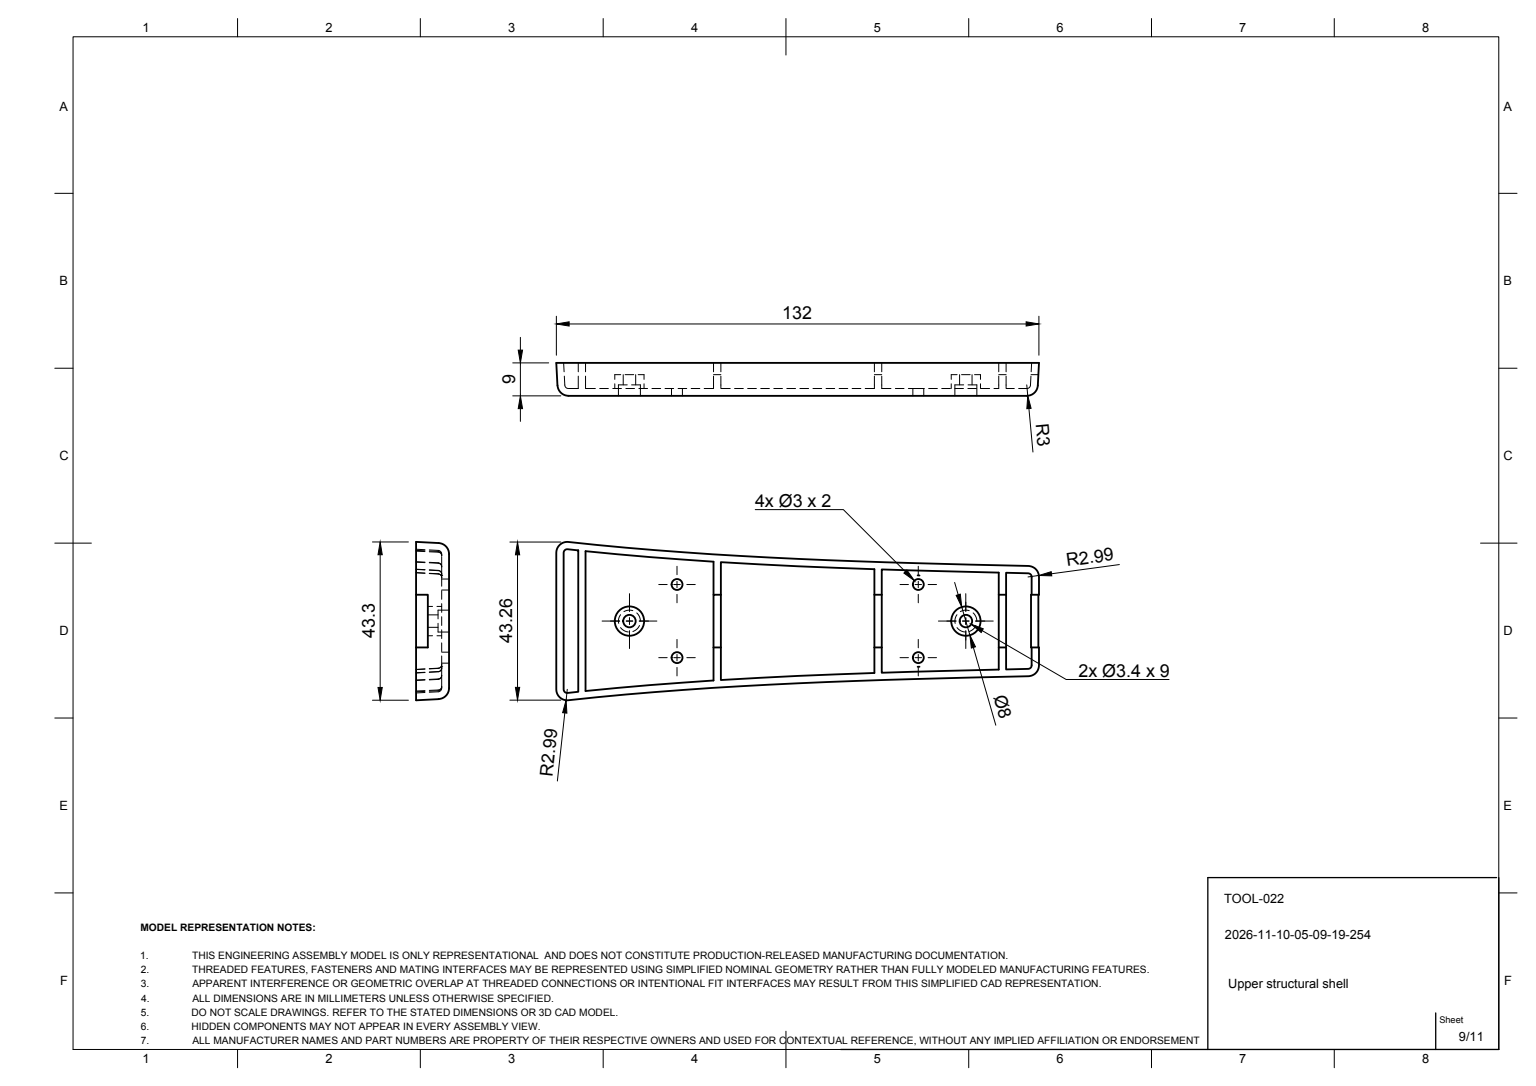
ISO-10303-21;
HEADER;
/* Generated by software containing ST-Developer
 * from STEP Tools, Inc. (www.steptools.com) 
 */

FILE_DESCRIPTION(
/* description */ (''),
/* implementation_level */ '2;1');

FILE_NAME(
/* name */ 'Upper structural shell.step',
/* time_stamp */ '2026-11-10T08:27:36-08:00',
/* author */ (''),
/* organization */ (''),
/* preprocessor_version */ 'ST-DEVELOPER v20.2',
/* originating_system */ 'Autodesk Translation Framework v15.17.0.0',
/* authorisation */ '');

FILE_SCHEMA (('AUTOMOTIVE_DESIGN { 1 0 10303 214 3 1 1 }'));
ENDSEC;

DATA;
#10=MECHANICAL_DESIGN_GEOMETRIC_PRESENTATION_REPRESENTATION('',(#570),#19090);
#76=SPHERICAL_SURFACE('',#7106,0.0999999999999999);
#77=SPHERICAL_SURFACE('',#7109,0.0999999999999997);
#78=SPHERICAL_SURFACE('',#7113,0.0999999999999998);
#79=SPHERICAL_SURFACE('',#7117,0.1);
#80=SPHERICAL_SURFACE('',#7122,0.3);
#81=SPHERICAL_SURFACE('',#7126,0.3);
#82=SPHERICAL_SURFACE('',#7130,0.3);
#83=SPHERICAL_SURFACE('',#7135,0.3);
#92=B_SPLINE_SURFACE_WITH_KNOTS('',3,3,((#10183,#10184,#10185,#10186),(#10187,
#10188,#10189,#10190),(#10191,#10192,#10193,#10194),(#10195,#10196,#10197,
#10198)),.UNSPECIFIED.,.F.,.F.,.F.,(4,4),(4,4),(0.0600191787356395,0.326709122771036),
(0.0105314009467253,0.683686938235975),.UNSPECIFIED.);
#93=B_SPLINE_SURFACE_WITH_KNOTS('',3,3,((#10203,#10204,#10205,#10206),(#10207,
#10208,#10209,#10210),(#10211,#10212,#10213,#10214),(#10215,#10216,#10217,
#10218)),.UNSPECIFIED.,.F.,.F.,.F.,(4,4),(4,4),(0.0251675824878611,0.0470055662028096),
(0.0103663370325175,0.682341693918943),.UNSPECIFIED.);
#94=B_SPLINE_SURFACE_WITH_KNOTS('',3,3,((#10228,#10229,#10230,#10231),(#10232,
#10233,#10234,#10235),(#10236,#10237,#10238,#10239),(#10240,#10241,#10242,
#10243),(#10244,#10245,#10246,#10247)),.UNSPECIFIED.,.F.,.F.,.F.,(4,1,4),
(4,4),(0.,0.571428571428571,1.),(0.796205213256333,4.31873271634551),
 .UNSPECIFIED.);
#95=B_SPLINE_SURFACE_WITH_KNOTS('',3,3,((#10252,#10253,#10254,#10255),(#10256,
#10257,#10258,#10259),(#10260,#10261,#10262,#10263),(#10264,#10265,#10266,
#10267),(#10268,#10269,#10270,#10271)),.UNSPECIFIED.,.F.,.F.,.F.,(4,1,4),
(4,4),(0.,0.571428571428571,1.),(0.335767855111383,0.605460332260614),
 .UNSPECIFIED.);
#96=B_SPLINE_SURFACE_WITH_KNOTS('',3,3,((#10290,#10291,#10292,#10293),(#10294,
#10295,#10296,#10297),(#10298,#10299,#10300,#10301),(#10302,#10303,#10304,
#10305),(#10306,#10307,#10308,#10309)),.UNSPECIFIED.,.F.,.F.,.F.,(4,1,4),
(4,4),(0.,0.571428571428571,1.),(8.8675541747208,12.3900816778099),
 .UNSPECIFIED.);
#97=B_SPLINE_SURFACE_WITH_KNOTS('',3,3,((#10314,#10315,#10316,#10317),(#10318,
#10319,#10320,#10321),(#10322,#10323,#10324,#10325),(#10326,#10327,#10328,
#10329)),.UNSPECIFIED.,.F.,.F.,.F.,(4,4),(4,4),(0.673290877228964,0.939980821264432),
(0.010531400969624,0.683686938235975),.UNSPECIFIED.);
#98=B_SPLINE_SURFACE_WITH_KNOTS('',3,3,((#10330,#10331,#10332,#10333),(#10334,
#10335,#10336,#10337),(#10338,#10339,#10340,#10341),(#10342,#10343,#10344,
#10345)),.UNSPECIFIED.,.F.,.F.,.F.,(4,4),(4,4),(0.952994433797115,0.974832417512139),
(0.0103663370325174,0.682341693895801),.UNSPECIFIED.);
#99=B_SPLINE_SURFACE_WITH_KNOTS('',3,3,((#10429,#10430,#10431,#10432),(#10433,
#10434,#10435,#10436),(#10437,#10438,#10439,#10440),(#10441,#10442,#10443,
#10444)),.UNSPECIFIED.,.F.,.F.,.F.,(4,4),(4,4),(0.341076481775573,0.660379921919131),
(0.0113804342297301,0.684288445414502),.UNSPECIFIED.);
#100=B_SPLINE_SURFACE_WITH_KNOTS('',3,3,((#10449,#10450,#10451,#10452),
(#10453,#10454,#10455,#10456),(#10457,#10458,#10459,#10460),(#10461,#10462,
#10463,#10464),(#10465,#10466,#10467,#10468)),.UNSPECIFIED.,.F.,.F.,.F.,
(4,1,4),(4,4),(0.,0.571428571428571,1.),(4.5128966022766,8.72381854299666),
 .UNSPECIFIED.);
#101=B_SPLINE_SURFACE_WITH_KNOTS('',3,3,((#10478,#10479,#10480,#10481),
(#10482,#10483,#10484,#10485),(#10486,#10487,#10488,#10489),(#10490,#10491,
#10492,#10493),(#10494,#10495,#10496,#10497)),.UNSPECIFIED.,.F.,.F.,.F.,
(4,1,4),(4,4),(0.,0.571428571428571,1.),(4.46246834806959,8.67339028878965),
 .UNSPECIFIED.);
#102=B_SPLINE_SURFACE_WITH_KNOTS('',3,3,((#10502,#10503,#10504,#10505),
(#10506,#10507,#10508,#10509),(#10510,#10511,#10512,#10513),(#10514,#10515,
#10516,#10517)),.UNSPECIFIED.,.F.,.F.,.F.,(4,4),(4,4),(0.33962007808087,
0.658923518224427),(0.0113804342297301,0.68428844541339),.UNSPECIFIED.);
#103=B_SPLINE_SURFACE_WITH_KNOTS('',3,3,((#10589,#10590,#10591,#10592),
(#10593,#10594,#10595,#10596),(#10597,#10598,#10599,#10600),(#10601,#10602,
#10603,#10604)),.UNSPECIFIED.,.F.,.F.,.F.,(4,4),(4,4),(0.67474627241906,
0.91907102854965),(0.0117551961069005,0.684448842095107),.UNSPECIFIED.);
#104=B_SPLINE_SURFACE_WITH_KNOTS('',3,3,((#10609,#10610,#10611,#10612),
(#10613,#10614,#10615,#10616),(#10617,#10618,#10619,#10620),(#10621,#10622,
#10623,#10624),(#10625,#10626,#10627,#10628)),.UNSPECIFIED.,.F.,.F.,.F.,
(4,1,4),(4,4),(0.,0.571428571428571,1.),(8.92068531110742,12.1251256661408),
 .UNSPECIFIED.);
#105=B_SPLINE_SURFACE_WITH_KNOTS('',3,3,((#10629,#10630,#10631,#10632),
(#10633,#10634,#10635,#10636),(#10637,#10638,#10639,#10640),(#10641,#10642,
#10643,#10644),(#10645,#10646,#10647,#10648)),.UNSPECIFIED.,.F.,.F.,.F.,
(4,1,4),(4,4),(0.,0.571428571428571,1.),(1.06116122492545,4.26560157995882),
 .UNSPECIFIED.);
#106=B_SPLINE_SURFACE_WITH_KNOTS('',3,3,((#10653,#10654,#10655,#10656),
(#10657,#10658,#10659,#10660),(#10661,#10662,#10663,#10664),(#10665,#10666,
#10667,#10668)),.UNSPECIFIED.,.F.,.F.,.F.,(4,4),(4,4),(0.0809289714503497,
0.325253727580939),(0.011755196108102,0.684448842095106),.UNSPECIFIED.);
#107=B_SPLINE_SURFACE_WITH_KNOTS('',3,3,((#10743,#10744,#10745,#10746),
(#10747,#10748,#10749,#10750),(#10751,#10752,#10753,#10754),(#10755,#10756,
#10757,#10758)),.UNSPECIFIED.,.F.,.F.,.F.,(4,4),(4,4),(0.932204931312898,
0.977820042778932),(0.0118590921259657,0.68448768567755),.UNSPECIFIED.);
#108=B_SPLINE_SURFACE_WITH_KNOTS('',3,3,((#10768,#10769,#10770,#10771),
(#10772,#10773,#10774,#10775),(#10776,#10777,#10778,#10779),(#10780,#10781,
#10782,#10783),(#10784,#10785,#10786,#10787)),.UNSPECIFIED.,.F.,.F.,.F.,
(4,1,4),(4,4),(0.,0.571428571428571,1.),(12.3228618033436,12.893479658151),
 .UNSPECIFIED.);
#109=B_SPLINE_SURFACE_WITH_KNOTS('',3,3,((#10801,#10802,#10803,#10804),
(#10805,#10806,#10807,#10808),(#10809,#10810,#10811,#10812),(#10813,#10814,
#10815,#10816)),.UNSPECIFIED.,.F.,.F.,.F.,(4,4),(4,4),(0.0221799572210682,
0.0677950686870383),(0.0118590921467069,0.68448768567755),.UNSPECIFIED.);
#110=B_SPLINE_SURFACE_WITH_KNOTS('',3,3,((#10826,#10827,#10828,#10829),
(#10830,#10831,#10832,#10833),(#10834,#10835,#10836,#10837),(#10838,#10839,
#10840,#10841),(#10842,#10843,#10844,#10845)),.UNSPECIFIED.,.F.,.F.,.F.,
(4,1,4),(4,4),(0.,0.571428571428571,1.),(0.29280723291527,0.863425087722636),
 .UNSPECIFIED.);
#111=B_SPLINE_SURFACE_WITH_KNOTS('',3,3,((#10859,#10860,#10861,#10862),
(#10863,#10864,#10865,#10866),(#10867,#10868,#10869,#10870),(#10871,#10872,
#10873,#10874),(#10875,#10876,#10877,#10878)),.UNSPECIFIED.,.F.,.F.,.F.,
(4,1,4),(4,4),(0.,0.571428571428571,1.),(0.00866835330220971,0.617725317592517),
 .UNSPECIFIED.);
#112=B_SPLINE_SURFACE_WITH_KNOTS('',3,3,((#10885,#10886,#10887,#10888),
(#10889,#10890,#10891,#10892),(#10893,#10894,#10895,#10896),(#10897,#10898,
#10899,#10900),(#10901,#10902,#10903,#10904),(#10905,#10906,#10907,#10908)),
 .UNSPECIFIED.,.F.,.F.,.F.,(4,1,1,4),(4,4),(0.,0.285714285714286,0.571428571428571,
1.),(0.00654045782928703,0.615688454110788),.UNSPECIFIED.);
#113=B_SPLINE_SURFACE_WITH_KNOTS('',3,3,((#10913,#10914,#10915,#10916),
(#10917,#10918,#10919,#10920),(#10921,#10922,#10923,#10924),(#10925,#10926,
#10927,#10928),(#10929,#10930,#10931,#10932),(#10933,#10934,#10935,#10936)),
 .UNSPECIFIED.,.F.,.F.,.F.,(4,1,1,4),(4,4),(0.,0.285714285714286,0.571428571428571,
1.),(0.00659363931523289,0.615688454110787),.UNSPECIFIED.);
#114=B_SPLINE_SURFACE_WITH_KNOTS('',3,3,((#10941,#10942,#10943,#10944),
(#10945,#10946,#10947,#10948),(#10949,#10950,#10951,#10952),(#10953,#10954,
#10955,#10956),(#10957,#10958,#10959,#10960)),.UNSPECIFIED.,.F.,.F.,.F.,
(4,1,4),(4,4),(0.,0.571428571428571,1.),(12.5808265588057,12.8505190359549),
 .UNSPECIFIED.);
#115=B_SPLINE_SURFACE_WITH_KNOTS('',3,3,((#10961,#10962,#10963,#10964),
(#10965,#10966,#10967,#10968),(#10969,#10970,#10971,#10972),(#10973,#10974,
#10975,#10976),(#10977,#10978,#10979,#10980)),.UNSPECIFIED.,.F.,.F.,.F.,
(4,1,4),(4,4),(0.,0.571428571428571,1.),(0.00865878607617127,0.617725317592517),
 .UNSPECIFIED.);
#116=B_SPLINE_SURFACE_WITH_KNOTS('',3,3,((#11006,#11007,#11008,#11009),
(#11010,#11011,#11012,#11013),(#11014,#11015,#11016,#11017),(#11018,#11019,
#11020,#11021),(#11022,#11023,#11024,#11025)),.UNSPECIFIED.,.F.,.F.,.F.,
(4,1,4),(4,4),(0.,0.571428571428571,1.),(-0.00615755989250974,0.617725317592517),
 .UNSPECIFIED.);
#117=B_SPLINE_SURFACE_WITH_KNOTS('',3,3,((#11044,#11045,#11046,#11047,#11048),
(#11049,#11050,#11051,#11052,#11053),(#11054,#11055,#11056,#11057,#11058),
(#11059,#11060,#11061,#11062,#11063),(#11064,#11065,#11066,#11067,#11068)),
 .UNSPECIFIED.,.F.,.F.,.F.,(4,1,4),(4,1,4),(0.,0.571428571428571,1.),(0.335767855111383,
5.71764434212835,12.893479658151),.UNSPECIFIED.);
#118=B_SPLINE_SURFACE_WITH_KNOTS('',3,3,((#11079,#11080,#11081,#11082),
(#11083,#11084,#11085,#11086),(#11087,#11088,#11089,#11090),(#11091,#11092,
#11093,#11094),(#11095,#11096,#11097,#11098),(#11099,#11100,#11101,#11102)),
 .UNSPECIFIED.,.F.,.F.,.F.,(4,1,1,4),(4,4),(0.,0.285714285714286,0.571428571428571,
1.),(-0.00844595120920508,0.615688454110788),.UNSPECIFIED.);
#119=B_SPLINE_SURFACE_WITH_KNOTS('',3,3,((#11111,#11112,#11113,#11114),
(#11115,#11116,#11117,#11118),(#11119,#11120,#11121,#11122),(#11123,#11124,
#11125,#11126),(#11127,#11128,#11129,#11130),(#11131,#11132,#11133,#11134)),
 .UNSPECIFIED.,.F.,.F.,.F.,(4,1,1,4),(4,4),(0.,0.285714285714286,0.571428571428571,
1.),(-0.00828643285111643,0.615688454110787),.UNSPECIFIED.);
#120=B_SPLINE_SURFACE_WITH_KNOTS('',3,3,((#11143,#11144,#11145,#11146,#11147),
(#11148,#11149,#11150,#11151,#11152),(#11153,#11154,#11155,#11156,#11157),
(#11158,#11159,#11160,#11161,#11162),(#11163,#11164,#11165,#11166,#11167)),
 .UNSPECIFIED.,.F.,.F.,.F.,(4,1,4),(4,1,4),(0.,0.571428571428571,1.),(0.29280723291527,
7.4686425489379,12.8505190359549),.UNSPECIFIED.);
#121=B_SPLINE_SURFACE_WITH_KNOTS('',3,3,((#11178,#11179,#11180,#11181),
(#11182,#11183,#11184,#11185),(#11186,#11187,#11188,#11189),(#11190,#11191,
#11192,#11193),(#11194,#11195,#11196,#11197)),.UNSPECIFIED.,.F.,.F.,.F.,
(4,1,4),(4,4),(0.,0.571428571428571,1.),(-0.0061862132014275,0.617725317592517),
 .UNSPECIFIED.);
#122=B_SPLINE_SURFACE_WITH_KNOTS('',3,3,((#11206,#11207,#11208,#11209),
(#11210,#11211,#11212,#11213),(#11214,#11215,#11216,#11217),(#11218,#11219,
#11220,#11221)),.UNSPECIFIED.,.F.,.F.,.F.,(4,4),(4,4),(0.025165545222094,
0.977821881680028),(0.,0.68448768567755),.UNSPECIFIED.);
#123=B_SPLINE_SURFACE_WITH_KNOTS('',3,3,((#11224,#11225,#11226,#11227),
(#11228,#11229,#11230,#11231),(#11232,#11233,#11234,#11235),(#11236,#11237,
#11238,#11239)),.UNSPECIFIED.,.F.,.F.,.F.,(4,4),(4,4),(0.0221781183199723,
0.974834454777906),(0.,0.68448768567755),.UNSPECIFIED.);
#172=B_SPLINE_CURVE_WITH_KNOTS('',3,(#9197,#9198,#9199,#9200),
 .UNSPECIFIED.,.F.,.F.,(4,4),(3.28016616408593,4.26236080300681),
 .UNSPECIFIED.);
#173=B_SPLINE_CURVE_WITH_KNOTS('',3,(#9204,#9205,#9206,#9207),
 .UNSPECIFIED.,.F.,.F.,(4,4),(8.92392608805945,9.90612072688831),
 .UNSPECIFIED.);
#174=B_SPLINE_CURVE_WITH_KNOTS('',3,(#9209,#9210,#9211,#9212,#9213,#9214,
#9215,#9216,#9217,#9218,#9219,#9220,#9221,#9222,#9223,#9224,#9225,#9226,
#9227),.UNSPECIFIED.,.F.,.F.,(4,3,3,3,3,3,4),(-0.050768112872884,-0.0388528786649772,
-0.0311058171716578,-0.0259830388669653,-0.0210744122964195,-0.0143837148934404,
0.),.UNSPECIFIED.);
#175=B_SPLINE_CURVE_WITH_KNOTS('',3,(#9229,#9230,#9231,#9232),
 .UNSPECIFIED.,.F.,.F.,(4,4),(9.9568018127159,12.1251256661408),
 .UNSPECIFIED.);
#176=B_SPLINE_CURVE_WITH_KNOTS('',3,(#9236,#9237,#9238,#9239),
 .UNSPECIFIED.,.F.,.F.,(4,4),(1.06116122492545,3.22948508825557),
 .UNSPECIFIED.);
#177=B_SPLINE_CURVE_WITH_KNOTS('',3,(#9240,#9241,#9242,#9243,#9244,#9245,
#9246,#9247,#9248,#9249,#9250,#9251,#9252,#9253,#9254,#9255,#9256,#9257,
#9258),.UNSPECIFIED.,.F.,.F.,(4,3,3,3,3,3,4),(-0.0507681129736439,-0.0388528772897764,
-0.0311058147321604,-0.0259830361493327,-0.0210744097201194,-0.0143837130754026,
-9.90506278315E-9),.UNSPECIFIED.);
#178=B_SPLINE_CURVE_WITH_KNOTS('',3,(#9406,#9407,#9408,#9409,#9410,#9411),
 .UNSPECIFIED.,.F.,.F.,(4,2,4),(-0.605566356596631,-0.303329629920269,-0.000148729590407126),
 .UNSPECIFIED.);
#179=B_SPLINE_CURVE_WITH_KNOTS('',3,(#9413,#9414,#9415,#9416,#9417,#9418,
#9419,#9420,#9421,#9422,#9423,#9424,#9425,#9426,#9427,#9428,#9429,#9430,
#9431,#9432,#9433,#9434,#9435,#9436,#9437,#9438,#9439,#9440),
 .UNSPECIFIED.,.F.,.F.,(4,3,3,3,3,3,3,3,3,4),(-0.153210533292091,-0.129383071834804,
-0.117098895005168,-0.0931297672424715,-0.0778761857300216,-0.065564095006876,
-0.0417435583396367,-0.038874550231651,-0.0150983388519663,0.),
 .UNSPECIFIED.);
#180=B_SPLINE_CURVE_WITH_KNOTS('',3,(#9444,#9445,#9446,#9447,#9448,#9449,
#9450,#9451,#9452,#9453,#9454,#9455,#9456,#9457,#9458,#9459,#9460,#9461,
#9462,#9463,#9464,#9465,#9466,#9467,#9468,#9469,#9470,#9471),
 .UNSPECIFIED.,.F.,.F.,(4,3,3,3,3,3,3,3,3,4),(-0.153244081227051,-0.129493605146206,
-0.117970006482883,-0.0941492904140308,-0.0876825809854227,-0.078828741443105,
-0.0548877675055393,-0.0394694906046094,-0.0155984926894347,0.),
 .UNSPECIFIED.);
#181=B_SPLINE_CURVE_WITH_KNOTS('',3,(#9472,#9473,#9474,#9475,#9476,#9477),
 .UNSPECIFIED.,.F.,.F.,(4,2,4),(-0.606539490527658,-0.303329031627741,-0.00112184825655631),
 .UNSPECIFIED.);
#182=B_SPLINE_CURVE_WITH_KNOTS('',3,(#9482,#9483,#9484,#9485,#9486,#9487),
 .UNSPECIFIED.,.F.,.F.,(4,2,4),(-0.606785247764818,-0.303663188081886,-0.00088649083675002),
 .UNSPECIFIED.);
#183=B_SPLINE_CURVE_WITH_KNOTS('',3,(#9489,#9490,#9491,#9492,#9493,#9494,
#9495,#9496,#9497,#9498,#9499,#9500,#9501,#9502,#9503,#9504,#9505,#9506,
#9507,#9508,#9509,#9510,#9511,#9512,#9513,#9514,#9515,#9516),
 .UNSPECIFIED.,.F.,.F.,(4,3,3,3,3,3,3,3,3,4),(-0.15258577077829,-0.128839317352572,
-0.117158786685373,-0.0932148261566644,-0.0780319390000633,-0.0653676349965338,
-0.0415665498371782,-0.0389909618069961,-0.0152059030050533,0.),
 .UNSPECIFIED.);
#184=B_SPLINE_CURVE_WITH_KNOTS('',3,(#9520,#9521,#9522,#9523,#9524,#9525,
#9526,#9527,#9528,#9529,#9530,#9531,#9532,#9533,#9534,#9535,#9536,#9537,
#9538,#9539,#9540,#9541,#9542,#9543,#9544,#9545,#9546,#9547),
 .UNSPECIFIED.,.F.,.F.,(4,3,3,3,3,3,3,3,3,4),(-0.152596853546747,-0.128825864440686,
-0.115507515430042,-0.0917263797372463,-0.0872428123353572,-0.0783995504057471,
-0.0544835945915644,-0.0392209901554083,-0.0154275313391792,0.),
 .UNSPECIFIED.);
#185=B_SPLINE_CURVE_WITH_KNOTS('',3,(#9549,#9550,#9551,#9552,#9553,#9554),
 .UNSPECIFIED.,.F.,.F.,(4,2,4),(-0.606440835737524,-0.303663090452391,-0.000542069086802599),
 .UNSPECIFIED.);
#186=B_SPLINE_CURVE_WITH_KNOTS('',3,(#9560,#9561,#9562,#9563,#9564,#9565),
 .UNSPECIFIED.,.F.,.F.,(4,2,4),(-0.607379220946441,-0.303761646676304,-0.00124422999587004),
 .UNSPECIFIED.);
#187=B_SPLINE_CURVE_WITH_KNOTS('',3,(#9567,#9568,#9569,#9570,#9571,#9572,
#9573,#9574,#9575,#9576,#9577,#9578,#9579,#9580,#9581,#9582,#9583,#9584,
#9585,#9586,#9587,#9588,#9589,#9590,#9591,#9592,#9593,#9594),
 .UNSPECIFIED.,.F.,.F.,(4,3,3,3,3,3,3,3,3,4),(-0.152287640102895,-0.128554450486317,
-0.115193035178751,-0.0912770810520543,-0.0781028969167454,-0.0652733399726575,
-0.0414820896655672,-0.0390446621366508,-0.0152552334863041,0.),
 .UNSPECIFIED.);
#188=B_SPLINE_CURVE_WITH_KNOTS('',3,(#9598,#9599,#9600,#9601,#9602,#9603,
#9604,#9605,#9606,#9607,#9608,#9609,#9610,#9611,#9612,#9613,#9614,#9615,
#9616,#9617,#9618,#9619,#9620,#9621,#9622,#9623,#9624,#9625),
 .UNSPECIFIED.,.F.,.F.,(4,3,3,3,3,3,3,3,3,4),(-0.152291020205185,-0.128517753946702,
-0.115248901231919,-0.0914807886786037,-0.0870359119466785,-0.0782017654295232,
-0.054298407767766,-0.03910658747416,-0.0153486482327859,0.),
 .UNSPECIFIED.);
#189=B_SPLINE_CURVE_WITH_KNOTS('',3,(#9627,#9628,#9629,#9630,#9631,#9632),
 .UNSPECIFIED.,.F.,.F.,(4,2,4),(-0.606279550122448,-0.303761677523001,-0.000144559171857295),
 .UNSPECIFIED.);
#190=B_SPLINE_CURVE_WITH_KNOTS('',3,(#9638,#9639,#9640,#9641,#9642,#9643),
 .UNSPECIFIED.,.F.,.F.,(4,2,4),(-0.607536685592867,-0.303784463250135,-0.00133982193348342),
 .UNSPECIFIED.);
#191=B_SPLINE_CURVE_WITH_KNOTS('',3,(#9644,#9645,#9646,#9647,#9648,#9649,
#9650,#9651,#9652,#9653,#9654,#9655,#9656,#9657,#9658,#9659,#9660,#9661,
#9662,#9663,#9664,#9665,#9666,#9667,#9668,#9669,#9670,#9671),
 .UNSPECIFIED.,.F.,.F.,(4,3,3,3,3,3,3,3,3,4),(-0.152217684890348,-0.128490376540845,
-0.11516578527262,-0.091253137134092,-0.0781160865160423,-0.0652495101170982,
-0.0414606291875136,-0.0390546905501479,-0.015263466236765,0.),
 .UNSPECIFIED.);
#192=B_SPLINE_CURVE_WITH_KNOTS('',3,(#9673,#9674,#9675,#9676,#9677,#9678,
#9679,#9680,#9681,#9682,#9683,#9684,#9685,#9686,#9687,#9688,#9689,#9690,
#9691,#9692,#9693,#9694,#9695,#9696,#9697,#9698,#9699,#9700),
 .UNSPECIFIED.,.F.,.F.,(4,3,3,3,3,3,3,3,3,4),(-0.152219351639196,-0.128444680332832,
-0.115193337419806,-0.0914284185691762,-0.0869890032859244,-0.0781648487722283,
-0.0542647883944502,-0.0390852411900305,-0.0153331469286526,0.),
 .UNSPECIFIED.);
#193=B_SPLINE_CURVE_WITH_KNOTS('',3,(#9702,#9703,#9704,#9705,#9706,#9707),
 .UNSPECIFIED.,.F.,.F.,(4,2,4),(-0.606231877025315,-0.303784501204342,-3.50089943914611E-5),
 .UNSPECIFIED.);
#194=B_SPLINE_CURVE_WITH_KNOTS('',3,(#9713,#9714,#9715,#9716),
 .UNSPECIFIED.,.F.,.F.,(4,4),(0.0108333608245492,0.617725317592517),
 .UNSPECIFIED.);
#195=B_SPLINE_CURVE_WITH_KNOTS('',3,(#9720,#9721,#9722,#9723),
 .UNSPECIFIED.,.F.,.F.,(4,4),(-0.617725317592517,-0.0108333608245492),
 .UNSPECIFIED.);
#196=B_SPLINE_CURVE_WITH_KNOTS('',3,(#9726,#9727,#9728,#9729),
 .UNSPECIFIED.,.F.,.F.,(4,4),(8.65483889175297,12.1899094612697),
 .UNSPECIFIED.);
#197=B_SPLINE_CURVE_WITH_KNOTS('',3,(#9730,#9731,#9732,#9733),
 .UNSPECIFIED.,.F.,.F.,(4,4),(0.491886782059505,4.00844302274363),
 .UNSPECIFIED.);
#198=B_SPLINE_CURVE_WITH_KNOTS('',3,(#9736,#9737,#9738,#9739,#9740,#9741,
#9742,#9743,#9744,#9745),.UNSPECIFIED.,.F.,.F.,(4,3,3,4),(4.20909064274042,
6.3236533433415,8.26419514194387,8.41669725637478),.UNSPECIFIED.);
#199=B_SPLINE_CURVE_WITH_KNOTS('',3,(#9748,#9749,#9750,#9751),
 .UNSPECIFIED.,.F.,.F.,(4,4),(8.61714174069208,11.8187712274298),
 .UNSPECIFIED.);
#200=B_SPLINE_CURVE_WITH_KNOTS('',3,(#9755,#9756,#9757,#9758),
 .UNSPECIFIED.,.F.,.F.,(4,4),(12.0182076143484,12.6179302061492),
 .UNSPECIFIED.);
#201=B_SPLINE_CURVE_WITH_KNOTS('',3,(#9759,#9760,#9761,#9762,#9763,#9764,
#9765,#9766,#9767,#9768,#9769,#9770,#9771,#9772,#9773,#9774,#9775,#9776,
#9777,#9778,#9779,#9780,#9781,#9782,#9783,#9784,#9785,#9786),
 .UNSPECIFIED.,.F.,.F.,(4,3,3,3,3,3,3,3,3,4),(0.,0.023812730958415,0.0390943730497349,
0.0628727645281949,0.0664866407211859,0.0780895647789142,0.102003044086093,
0.117056568347941,0.14081843048439,0.155095961761698),.UNSPECIFIED.);
#202=B_SPLINE_CURVE_WITH_KNOTS('',3,(#9790,#9791,#9792,#9793,#9794,#9795,
#9796,#9797,#9798,#9799,#9800,#9801,#9802,#9803,#9804,#9805,#9806,#9807,
#9808,#9809,#9810,#9811,#9812,#9813,#9814,#9815,#9816,#9817,#9818,#9819,
#9820,#9821,#9822,#9823,#9824,#9825,#9826),.UNSPECIFIED.,.F.,.F.,(4,3,3,
3,3,3,3,3,3,3,3,3,4),(0.,0.0535193130531386,0.107740084455895,0.117281563739951,
0.171478196787188,0.199460035548543,0.234266327019636,0.287962832542679,
0.34249270416273,0.351167719367162,0.408228095477446,0.46132246935065,0.46528847158773),
 .UNSPECIFIED.);
#203=B_SPLINE_CURVE_WITH_KNOTS('',3,(#9828,#9829,#9830,#9831),
 .UNSPECIFIED.,.F.,.F.,(4,4),(0.0221781183199723,0.974834454777906),
 .UNSPECIFIED.);
#204=B_SPLINE_CURVE_WITH_KNOTS('',3,(#9833,#9834,#9835,#9836,#9837,#9838,
#9839,#9840,#9841,#9842,#9843,#9844,#9845,#9846,#9847,#9848,#9849,#9850,
#9851,#9852,#9853,#9854,#9855,#9856,#9857,#9858,#9859,#9860,#9861,#9862,
#9863,#9864,#9865,#9866,#9867,#9868,#9869,#9870,#9871,#9872,#9873,#9874,
#9875),.UNSPECIFIED.,.F.,.F.,(4,3,3,3,3,3,3,3,3,3,3,3,3,3,4),(0.,0.0533317239385299,
0.107762434368039,0.117305236535198,0.171635266834242,0.216430402805854,
0.234303130921432,0.288010415584935,0.341932185058889,0.351200358601802,
0.360578786332496,0.414653942238971,0.427906071157934,0.482008506259547,
0.504658879840573),.UNSPECIFIED.);
#205=B_SPLINE_CURVE_WITH_KNOTS('',3,(#9879,#9880,#9881,#9882,#9883,#9884,
#9885,#9886,#9887,#9888,#9889,#9890,#9891,#9892,#9893,#9894,#9895,#9896,
#9897,#9898,#9899,#9900,#9901,#9902,#9903,#9904,#9905,#9906,#9907,#9908,
#9909,#9910,#9911,#9912,#9913,#9914,#9915,#9916,#9917,#9918,#9919,#9920,
#9921),.UNSPECIFIED.,.F.,.F.,(4,3,3,3,3,3,3,3,3,3,3,3,3,3,4),(0.,0.0533492049661439,
0.107791770949794,0.117401360885473,0.171729175646356,0.216477851539682,
0.234467324023732,0.288191829779795,0.342104640447882,0.351366010290958,
0.360619117109406,0.414688080797906,0.427993719046535,0.482081475021072,
0.504664253934307),.UNSPECIFIED.);
#206=B_SPLINE_CURVE_WITH_KNOTS('',3,(#9923,#9924,#9925,#9926),
 .UNSPECIFIED.,.F.,.F.,(4,4),(0.0251655452220943,0.977821881680028),
 .UNSPECIFIED.);
#207=B_SPLINE_CURVE_WITH_KNOTS('',3,(#9928,#9929,#9930,#9931,#9932,#9933,
#9934,#9935,#9936,#9937,#9938,#9939,#9940,#9941,#9942,#9943,#9944,#9945,
#9946,#9947,#9948,#9949,#9950,#9951,#9952,#9953,#9954,#9955,#9956,#9957,
#9958,#9959,#9960,#9961,#9962,#9963,#9964),.UNSPECIFIED.,.F.,.F.,(4,3,3,
3,3,3,3,3,3,3,3,3,4),(0.,0.053523079491772,0.107745541051727,0.117301531762597,
0.171497090450284,0.19946878868074,0.234298606923062,0.287998861062908,
0.34252758042597,0.351197710209308,0.408243668718811,0.4613343165756,0.465289627228313),
 .UNSPECIFIED.);
#208=B_SPLINE_CURVE_WITH_KNOTS('',3,(#9967,#9968,#9969,#9970,#9971,#9972,
#9973,#9974,#9975,#9976,#9977,#9978,#9979,#9980,#9981,#9982,#9983,#9984,
#9985,#9986,#9987,#9988,#9989,#9990,#9991,#9992,#9993,#9994),
 .UNSPECIFIED.,.F.,.F.,(4,3,3,3,3,3,3,3,3,4),(0.,0.0238139464176845,0.039101051769884,
0.0628789982206146,0.0664894862143964,0.0781003874493316,0.102014483019035,
0.11706667068295,0.140827139970411,0.155096347075245),.UNSPECIFIED.);
#209=B_SPLINE_CURVE_WITH_KNOTS('',3,(#9996,#9997,#9998,#9999),
 .UNSPECIFIED.,.F.,.F.,(4,4),(2.42791692093292E-5,0.602904494019558),
 .UNSPECIFIED.);
#210=B_SPLINE_CURVE_WITH_KNOTS('',3,(#10002,#10003,#10004,#10005),
 .UNSPECIFIED.,.F.,.F.,(4,4),(0.8033909285608,4.02187648095927),
 .UNSPECIFIED.);
#211=B_SPLINE_CURVE_WITH_KNOTS('',3,(#10008,#10009,#10010,#10011,#10012,
#10013,#10014,#10015,#10016,#10017),.UNSPECIFIED.,.F.,.F.,(4,3,3,4),(4.22337623295021,
6.17414866693447,6.32726315261627,8.45313487255185),.UNSPECIFIED.);
#212=B_SPLINE_CURVE_WITH_KNOTS('',3,(#10021,#10022,#10023,#10024),
 .UNSPECIFIED.,.F.,.F.,(4,4),(12.3921295467468,12.6843586902602),
 .UNSPECIFIED.);
#213=B_SPLINE_CURVE_WITH_KNOTS('',3,(#10026,#10027,#10028,#10029,#10030,
#10031,#10032,#10033,#10034,#10035,#10036,#10037,#10038,#10039,#10040,#10041,
#10042,#10043,#10044,#10045,#10046,#10047,#10048,#10049,#10050,#10051,#10052,
#10053,#10054,#10055,#10056,#10057,#10058,#10059),.UNSPECIFIED.,.F.,.F.,
(4,3,3,3,3,3,3,3,3,3,3,4),(0.,0.0238043957114055,0.0391346151758438,0.0629652053320384,
0.0721593756253901,0.0781571886687045,0.101948185591131,0.117123476992186,
0.12020682003633,0.142665945482357,0.166389927689249,0.168222194312373),
 .UNSPECIFIED.);
#214=B_SPLINE_CURVE_WITH_KNOTS('',3,(#10063,#10064,#10065,#10066,#10067,
#10068,#10069,#10070,#10071,#10072,#10073,#10074,#10075,#10076,#10077,#10078,
#10079,#10080,#10081,#10082,#10083,#10084,#10085,#10086,#10087,#10088,#10089,
#10090,#10091,#10092,#10093,#10094,#10095,#10096),.UNSPECIFIED.,.F.,.F.,
(4,3,3,3,3,3,3,3,3,3,3,4),(0.,0.023797882907907,0.039102479174454,0.0629340675289177,
0.0721439954475325,0.0781021576199648,0.101891255326939,0.117067721419617,
0.120193732390416,0.142636523050355,0.16636673084783,0.168220399847748),
 .UNSPECIFIED.);
#215=B_SPLINE_CURVE_WITH_KNOTS('',3,(#10098,#10099,#10100,#10101),
 .UNSPECIFIED.,.F.,.F.,(4,4),(2.71213177756024E-5,0.290725780256064),
 .UNSPECIFIED.);
#216=B_SPLINE_CURVE_WITH_KNOTS('',3,(#10111,#10112,#10113,#10114,#10115,
#10116),.UNSPECIFIED.,.F.,.F.,(4,2,4),(-0.6065913737563,-0.303324265158378,
-0.00121210420063977),.UNSPECIFIED.);
#217=B_SPLINE_CURVE_WITH_KNOTS('',3,(#10118,#10119,#10120,#10121,#10122,
#10123),.UNSPECIFIED.,.F.,.F.,(4,2,4),(-0.605468679705391,-0.303324901248498,
-8.9425867424664E-5),.UNSPECIFIED.);
#218=B_SPLINE_CURVE_WITH_KNOTS('',3,(#10125,#10126,#10127,#10128,#10129,
#10130,#10131,#10132,#10133,#10134,#10135,#10136,#10137,#10138,#10139,#10140,
#10141,#10142,#10143,#10144,#10145,#10146,#10147,#10148,#10149,#10150,#10151,
#10152),.UNSPECIFIED.,.F.,.F.,(4,3,3,3,3,3,3,3,3,4),(-0.153261590805415,
-0.129427422483982,-0.117093626371441,-0.093122524304512,-0.077863059046492,
-0.0655799937729104,-0.0417579003169496,-0.0388648221790391,-0.0150894148558222,
0.),.UNSPECIFIED.);
#219=B_SPLINE_CURVE_WITH_KNOTS('',3,(#10155,#10156,#10157,#10158,#10159,
#10160,#10161,#10162,#10163,#10164,#10165,#10166,#10167,#10168,#10169,#10170,
#10171,#10172,#10173,#10174,#10175,#10176,#10177,#10178,#10179,#10180,#10181,
#10182),.UNSPECIFIED.,.F.,.F.,(4,3,3,3,3,3,3,3,3,4),(-0.153296867786173,
-0.129546774976449,-0.118009772088948,-0.0941871764575653,-0.08771862273971,
-0.0788646444725944,-0.0549216410880561,-0.0394902966566095,-0.0156128557692252,
0.),.UNSPECIFIED.);
#220=B_SPLINE_CURVE_WITH_KNOTS('',3,(#10199,#10200,#10201,#10202),
 .UNSPECIFIED.,.F.,.F.,(4,4),(-4.3123055228435,-0.796205213256333),
 .UNSPECIFIED.);
#221=B_SPLINE_CURVE_WITH_KNOTS('',3,(#10220,#10221,#10222,#10223),
 .UNSPECIFIED.,.F.,.F.,(4,4),(-0.594853877716395,-0.335767855111383),
 .UNSPECIFIED.);
#222=B_SPLINE_CURVE_WITH_KNOTS('',3,(#10224,#10225,#10226,#10227),
 .UNSPECIFIED.,.F.,.F.,(4,4),(-0.615688454110788,-0.00935595183171186),
 .UNSPECIFIED.);
#223=B_SPLINE_CURVE_WITH_KNOTS('',3,(#10248,#10249,#10250,#10251),
 .UNSPECIFIED.,.F.,.F.,(4,4),(0.806548880270408,4.31873271634551),
 .UNSPECIFIED.);
#224=B_SPLINE_CURVE_WITH_KNOTS('',3,(#10273,#10274,#10275,#10276),
 .UNSPECIFIED.,.F.,.F.,(4,4),(0.335767855111383,0.605460332260614),
 .UNSPECIFIED.);
#225=B_SPLINE_CURVE_WITH_KNOTS('',3,(#10279,#10280,#10281,#10282),
 .UNSPECIFIED.,.F.,.F.,(4,4),(8.8675541747208,12.379738010796),
 .UNSPECIFIED.);
#226=B_SPLINE_CURVE_WITH_KNOTS('',3,(#10285,#10286,#10287,#10288),
 .UNSPECIFIED.,.F.,.F.,(4,4),(12.5808265588057,12.8505190359549),
 .UNSPECIFIED.);
#227=B_SPLINE_CURVE_WITH_KNOTS('',3,(#10310,#10311,#10312,#10313),
 .UNSPECIFIED.,.F.,.F.,(4,4),(-12.3900816778099,-8.87398136822274),
 .UNSPECIFIED.);
#228=B_SPLINE_CURVE_WITH_KNOTS('',3,(#10347,#10348,#10349,#10350),
 .UNSPECIFIED.,.F.,.F.,(4,4),(0.00935595183171174,0.615688454110787),
 .UNSPECIFIED.);
#229=B_SPLINE_CURVE_WITH_KNOTS('',3,(#10351,#10352,#10353,#10354),
 .UNSPECIFIED.,.F.,.F.,(4,4),(-12.8505190359549,-12.5914330133498),
 .UNSPECIFIED.);
#230=B_SPLINE_CURVE_WITH_KNOTS('',3,(#10357,#10358,#10359,#10360,#10361,
#10362),.UNSPECIFIED.,.F.,.F.,(4,2,4),(-0.606830654194234,-0.303665168982051,
-0.00091389508118378),.UNSPECIFIED.);
#231=B_SPLINE_CURVE_WITH_KNOTS('',3,(#10364,#10365,#10366,#10367,#10368,
#10369,#10370,#10371,#10372,#10373,#10374,#10375,#10376,#10377,#10378,#10379,
#10380,#10381,#10382,#10383,#10384,#10385,#10386,#10387,#10388,#10389,#10390,
#10391),.UNSPECIFIED.,.F.,.F.,(4,3,3,3,3,3,3,3,3,4),(-0.152562937837783,
-0.12881903955137,-0.117160811640917,-0.0932181166800446,-0.0780374575565173,
-0.0653603882662585,-0.0415602279441365,-0.0389951227734853,-0.0152093108541457,
0.),.UNSPECIFIED.);
#232=B_SPLINE_CURVE_WITH_KNOTS('',3,(#10395,#10396,#10397,#10398,#10399,
#10400,#10401,#10402,#10403,#10404,#10405,#10406,#10407,#10408,#10409,#10410,
#10411,#10412,#10413,#10414,#10415,#10416,#10417,#10418,#10419,#10420,#10421,
#10422),.UNSPECIFIED.,.F.,.F.,(4,3,3,3,3,3,3,3,3,4),(-0.152573286042523,
-0.128801685906155,-0.115487540236632,-0.091707628219999,-0.0872268515824704,
-0.07838422198738,-0.0544695788315335,-0.0392121213631617,-0.0154211067806385,
0.),.UNSPECIFIED.);
#233=B_SPLINE_CURVE_WITH_KNOTS('',3,(#10423,#10424,#10425,#10426,#10427,
#10428),.UNSPECIFIED.,.F.,.F.,(4,2,4),(-0.606417229744719,-0.30366508312326,
-0.000500462001714608),.UNSPECIFIED.);
#234=B_SPLINE_CURVE_WITH_KNOTS('',3,(#10445,#10446,#10447,#10448),
 .UNSPECIFIED.,.F.,.F.,(4,4),(-8.7204856127415,-4.5128966022766),
 .UNSPECIFIED.);
#235=B_SPLINE_CURVE_WITH_KNOTS('',3,(#10469,#10470,#10471,#10472),
 .UNSPECIFIED.,.F.,.F.,(4,4),(4.51913891174751,8.72381854299666),
 .UNSPECIFIED.);
#236=B_SPLINE_CURVE_WITH_KNOTS('',3,(#10474,#10475,#10476,#10477),
 .UNSPECIFIED.,.F.,.F.,(4,4),(4.46246834806959,8.66714797931881),
 .UNSPECIFIED.);
#237=B_SPLINE_CURVE_WITH_KNOTS('',3,(#10498,#10499,#10500,#10501),
 .UNSPECIFIED.,.F.,.F.,(4,4),(-8.67339028878965,-4.46580127832475),
 .UNSPECIFIED.);
#238=B_SPLINE_CURVE_WITH_KNOTS('',3,(#10520,#10521,#10522,#10523,#10524,
#10525),.UNSPECIFIED.,.F.,.F.,(4,2,4),(-0.607391644691745,-0.303762155877002,
-0.00125172564267001),.UNSPECIFIED.);
#239=B_SPLINE_CURVE_WITH_KNOTS('',3,(#10526,#10527,#10528,#10529,#10530,
#10531,#10532,#10533,#10534,#10535,#10536,#10537,#10538,#10539,#10540,#10541,
#10542,#10543,#10544,#10545,#10546,#10547,#10548,#10549,#10550,#10551,#10552,
#10553),.UNSPECIFIED.,.F.,.F.,(4,3,3,3,3,3,3,3,3,4),(-0.152281539067936,
-0.12854821222061,-0.115190816126163,-0.0912758856104041,-0.0781043161616985,
-0.0652713841318381,-0.0414808619979686,-0.039045740680325,-0.0152551599791835,
0.),.UNSPECIFIED.);
#240=B_SPLINE_CURVE_WITH_KNOTS('',3,(#10555,#10556,#10557,#10558,#10559,
#10560,#10561,#10562,#10563,#10564,#10565,#10566,#10567,#10568,#10569,#10570,
#10571,#10572,#10573,#10574,#10575,#10576,#10577,#10578,#10579,#10580,#10581,
#10582),.UNSPECIFIED.,.F.,.F.,(4,3,3,3,3,3,3,3,3,4),(-0.152284734818265,
-0.128510300097745,-0.115243636037359,-0.0914764658269932,-0.0870316758632336,
-0.078197793898112,-0.0542955901223581,-0.0391042908842167,-0.0153462458625635,
0.),.UNSPECIFIED.);
#241=B_SPLINE_CURVE_WITH_KNOTS('',3,(#10583,#10584,#10585,#10586,#10587,
#10588),.UNSPECIFIED.,.F.,.F.,(4,2,4),(-0.606273164239037,-0.303762187833104,
-0.000133245189939568),.UNSPECIFIED.);
#242=B_SPLINE_CURVE_WITH_KNOTS('',3,(#10605,#10606,#10607,#10608),
 .UNSPECIFIED.,.F.,.F.,(4,4),(-12.1227852464729,-8.92068531110742),
 .UNSPECIFIED.);
#243=B_SPLINE_CURVE_WITH_KNOTS('',3,(#10649,#10650,#10651,#10652),
 .UNSPECIFIED.,.F.,.F.,(4,4),(-4.26560157995882,-1.06350164459338),
 .UNSPECIFIED.);
#244=B_SPLINE_CURVE_WITH_KNOTS('',3,(#10671,#10672,#10673,#10674,#10675,
#10676),.UNSPECIFIED.,.F.,.F.,(4,2,4),(-0.607545900263938,-0.303784727094449,
-0.00134539382494125),.UNSPECIFIED.);
#245=B_SPLINE_CURVE_WITH_KNOTS('',3,(#10678,#10679,#10680,#10681,#10682,
#10683,#10684,#10685,#10686,#10687,#10688,#10689,#10690,#10691,#10692,#10693,
#10694,#10695,#10696,#10697,#10698,#10699,#10700,#10701,#10702,#10703,#10704,
#10705),.UNSPECIFIED.,.F.,.F.,(4,3,3,3,3,3,3,3,3,4),(-0.152214473108837,
-0.128485298747135,-0.115164309990209,-0.0912534321321267,-0.0781163092888813,
-0.0652482412471129,-0.0414606388666645,-0.0390548598067502,-0.0152611452145655,
0.),.UNSPECIFIED.);
#246=B_SPLINE_CURVE_WITH_KNOTS('',3,(#10709,#10710,#10711,#10712,#10713,
#10714,#10715,#10716,#10717,#10718,#10719,#10720,#10721,#10722,#10723,#10724,
#10725,#10726,#10727,#10728,#10729,#10730,#10731,#10732,#10733,#10734,#10735,
#10736),.UNSPECIFIED.,.F.,.F.,(4,3,3,3,3,3,3,3,3,4),(-0.152216110966007,
-0.128438825687404,-0.115191384846861,-0.0914281188167518,-0.0869870566155827,
-0.0781642271790374,-0.0542662950786889,-0.0390848818783988,-0.0153309789665,
0.),.UNSPECIFIED.);
#247=B_SPLINE_CURVE_WITH_KNOTS('',3,(#10737,#10738,#10739,#10740,#10741,
#10742),.UNSPECIFIED.,.F.,.F.,(4,2,4),(-0.606227037063105,-0.303784766192107,
-2.65251918123988E-5),.UNSPECIFIED.);
#248=B_SPLINE_CURVE_WITH_KNOTS('',3,(#10760,#10761,#10762,#10763),
 .UNSPECIFIED.,.F.,.F.,(4,4),(0.0107208554739345,0.617725317592517),
 .UNSPECIFIED.);
#249=B_SPLINE_CURVE_WITH_KNOTS('',3,(#10764,#10765,#10766,#10767),
 .UNSPECIFIED.,.F.,.F.,(4,4),(-12.893479658151,-12.3228618033436),
 .UNSPECIFIED.);
#250=B_SPLINE_CURVE_WITH_KNOTS('',3,(#10790,#10791,#10792,#10793),
 .UNSPECIFIED.,.F.,.F.,(4,4),(12.3251818525939,12.893479658151),
 .UNSPECIFIED.);
#251=B_SPLINE_CURVE_WITH_KNOTS('',3,(#10797,#10798,#10799,#10800),
 .UNSPECIFIED.,.F.,.F.,(4,4),(0.292807233425235,0.861105038472338),
 .UNSPECIFIED.);
#252=B_SPLINE_CURVE_WITH_KNOTS('',3,(#10818,#10819,#10820,#10821),
 .UNSPECIFIED.,.F.,.F.,(4,4),(-0.863425087722636,-0.29280723291527),
 .UNSPECIFIED.);
#253=B_SPLINE_CURVE_WITH_KNOTS('',3,(#10822,#10823,#10824,#10825),
 .UNSPECIFIED.,.F.,.F.,(4,4),(-0.617725317592517,-0.0107208554739345),
 .UNSPECIFIED.);
#254=B_SPLINE_CURVE_WITH_KNOTS('',3,(#10909,#10910,#10911,#10912),
 .UNSPECIFIED.,.F.,.F.,(4,4),(0.00878563933291533,0.615688454110788),
 .UNSPECIFIED.);
#255=B_SPLINE_CURVE_WITH_KNOTS('',3,(#10937,#10938,#10939,#10940),
 .UNSPECIFIED.,.F.,.F.,(4,4),(-0.615688454110787,-0.00878563933291527),
 .UNSPECIFIED.);
#256=B_SPLINE_CURVE_WITH_KNOTS('',3,(#11026,#11027,#11028,#11029),
 .UNSPECIFIED.,.F.,.F.,(4,4),(-9.62771529167128E-17,0.617725317592517),
 .UNSPECIFIED.);
#257=B_SPLINE_CURVE_WITH_KNOTS('',3,(#11030,#11031,#11032,#11033),
 .UNSPECIFIED.,.F.,.F.,(4,4),(-0.617725317592517,-0.000337488966422091),
 .UNSPECIFIED.);
#258=B_SPLINE_CURVE_WITH_KNOTS('',3,(#11069,#11070,#11071,#11072,#11073),
 .UNSPECIFIED.,.F.,.F.,(4,1,4),(-12.893479658151,-5.71764434212835,-0.335767855111383),
 .UNSPECIFIED.);
#259=B_SPLINE_CURVE_WITH_KNOTS('',3,(#11074,#11075,#11076,#11077,#11078),
 .UNSPECIFIED.,.F.,.F.,(4,1,4),(0.335767855111383,5.71764434212835,12.893479658151),
 .UNSPECIFIED.);
#260=B_SPLINE_CURVE_WITH_KNOTS('',3,(#11103,#11104,#11105,#11106),
 .UNSPECIFIED.,.F.,.F.,(4,4),(-0.00171041937131743,0.615688454110788),
 .UNSPECIFIED.);
#261=B_SPLINE_CURVE_WITH_KNOTS('',3,(#11107,#11108,#11109,#11110),
 .UNSPECIFIED.,.F.,.F.,(4,4),(-0.615688454110788,-3.98826847727851E-7),
 .UNSPECIFIED.);
#262=B_SPLINE_CURVE_WITH_KNOTS('',3,(#11135,#11136,#11137,#11138),
 .UNSPECIFIED.,.F.,.F.,(4,4),(3.98826847219577E-7,0.615688454110787),
 .UNSPECIFIED.);
#263=B_SPLINE_CURVE_WITH_KNOTS('',3,(#11139,#11140,#11141,#11142),
 .UNSPECIFIED.,.F.,.F.,(4,4),(-0.615688454110787,0.0017104193713176),
 .UNSPECIFIED.);
#264=B_SPLINE_CURVE_WITH_KNOTS('',3,(#11168,#11169,#11170,#11171,#11172),
 .UNSPECIFIED.,.F.,.F.,(4,1,4),(-12.8505190359549,-7.4686425489379,-0.29280723291527),
 .UNSPECIFIED.);
#265=B_SPLINE_CURVE_WITH_KNOTS('',3,(#11173,#11174,#11175,#11176,#11177),
 .UNSPECIFIED.,.F.,.F.,(4,1,4),(0.292807233425236,7.4686425489379,12.8505190359549),
 .UNSPECIFIED.);
#266=B_SPLINE_CURVE_WITH_KNOTS('',3,(#11198,#11199,#11200,#11201),
 .UNSPECIFIED.,.F.,.F.,(4,4),(0.000337488966421928,0.617725317592517),
 .UNSPECIFIED.);
#267=B_SPLINE_CURVE_WITH_KNOTS('',3,(#11202,#11203,#11204,#11205),
 .UNSPECIFIED.,.F.,.F.,(4,4),(-0.617725317592517,8.06646416329215E-17),
 .UNSPECIFIED.);
#550=SHAPE_REPRESENTATION_RELATIONSHIP('SRR','None',#19141,#560);
#560=ADVANCED_BREP_SHAPE_REPRESENTATION('',(#580),#19084);
#570=STYLED_ITEM('',(#19203),#580);
#580=MANIFOLD_SOLID_BREP('Body1',#6824);
#601=FACE_BOUND('',#1279,.T.);
#602=FACE_BOUND('',#1280,.T.);
#603=FACE_BOUND('',#1281,.T.);
#604=FACE_BOUND('',#1288,.T.);
#605=FACE_BOUND('',#1291,.T.);
#606=FACE_BOUND('',#1302,.T.);
#607=FACE_BOUND('',#1304,.T.);
#608=FACE_BOUND('',#1316,.T.);
#609=FACE_BOUND('',#1325,.T.);
#610=FACE_BOUND('',#1326,.T.);
#611=FACE_BOUND('',#1327,.T.);
#612=FACE_BOUND('',#1376,.T.);
#613=FACE_BOUND('',#1377,.T.);
#614=FACE_BOUND('',#1378,.T.);
#615=FACE_BOUND('',#1379,.T.);
#616=FACE_BOUND('',#1380,.T.);
#617=FACE_BOUND('',#1381,.T.);
#699=PLANE('',#7042);
#700=PLANE('',#7059);
#701=PLANE('',#7064);
#702=PLANE('',#7070);
#703=PLANE('',#7071);
#704=PLANE('',#7072);
#705=PLANE('',#7073);
#706=PLANE('',#7074);
#707=PLANE('',#7075);
#708=PLANE('',#7076);
#709=PLANE('',#7077);
#710=PLANE('',#7079);
#711=PLANE('',#7081);
#712=PLANE('',#7082);
#713=PLANE('',#7083);
#714=PLANE('',#7084);
#715=PLANE('',#7085);
#716=PLANE('',#7086);
#717=PLANE('',#7087);
#718=PLANE('',#7088);
#719=PLANE('',#7089);
#720=PLANE('',#7090);
#721=PLANE('',#7091);
#722=PLANE('',#7095);
#723=PLANE('',#7097);
#724=PLANE('',#7098);
#725=PLANE('',#7099);
#726=PLANE('',#7100);
#727=PLANE('',#7101);
#728=PLANE('',#7102);
#729=PLANE('',#7104);
#730=PLANE('',#7121);
#731=PLANE('',#7140);
#732=PLANE('',#7141);
#733=PLANE('',#7142);
#875=FACE_OUTER_BOUND('',#1278,.T.);
#876=FACE_OUTER_BOUND('',#1282,.T.);
#877=FACE_OUTER_BOUND('',#1283,.T.);
#878=FACE_OUTER_BOUND('',#1284,.T.);
#879=FACE_OUTER_BOUND('',#1285,.T.);
#880=FACE_OUTER_BOUND('',#1286,.T.);
#881=FACE_OUTER_BOUND('',#1287,.T.);
#882=FACE_OUTER_BOUND('',#1289,.T.);
#883=FACE_OUTER_BOUND('',#1290,.T.);
#884=FACE_OUTER_BOUND('',#1292,.T.);
#885=FACE_OUTER_BOUND('',#1293,.T.);
#886=FACE_OUTER_BOUND('',#1294,.T.);
#887=FACE_OUTER_BOUND('',#1295,.T.);
#888=FACE_OUTER_BOUND('',#1296,.T.);
#889=FACE_OUTER_BOUND('',#1297,.T.);
#890=FACE_OUTER_BOUND('',#1298,.T.);
#891=FACE_OUTER_BOUND('',#1299,.T.);
#892=FACE_OUTER_BOUND('',#1300,.T.);
#893=FACE_OUTER_BOUND('',#1301,.T.);
#894=FACE_OUTER_BOUND('',#1303,.T.);
#895=FACE_OUTER_BOUND('',#1305,.T.);
#896=FACE_OUTER_BOUND('',#1306,.T.);
#897=FACE_OUTER_BOUND('',#1307,.T.);
#898=FACE_OUTER_BOUND('',#1308,.T.);
#899=FACE_OUTER_BOUND('',#1309,.T.);
#900=FACE_OUTER_BOUND('',#1310,.T.);
#901=FACE_OUTER_BOUND('',#1311,.T.);
#902=FACE_OUTER_BOUND('',#1312,.T.);
#903=FACE_OUTER_BOUND('',#1313,.T.);
#904=FACE_OUTER_BOUND('',#1314,.T.);
#905=FACE_OUTER_BOUND('',#1315,.T.);
#906=FACE_OUTER_BOUND('',#1317,.T.);
#907=FACE_OUTER_BOUND('',#1318,.T.);
#908=FACE_OUTER_BOUND('',#1319,.T.);
#909=FACE_OUTER_BOUND('',#1320,.T.);
#910=FACE_OUTER_BOUND('',#1321,.T.);
#911=FACE_OUTER_BOUND('',#1322,.T.);
#912=FACE_OUTER_BOUND('',#1323,.T.);
#913=FACE_OUTER_BOUND('',#1324,.T.);
#914=FACE_OUTER_BOUND('',#1328,.T.);
#915=FACE_OUTER_BOUND('',#1329,.T.);
#916=FACE_OUTER_BOUND('',#1330,.T.);
#917=FACE_OUTER_BOUND('',#1331,.T.);
#918=FACE_OUTER_BOUND('',#1332,.T.);
#919=FACE_OUTER_BOUND('',#1333,.T.);
#920=FACE_OUTER_BOUND('',#1334,.T.);
#921=FACE_OUTER_BOUND('',#1335,.T.);
#922=FACE_OUTER_BOUND('',#1336,.T.);
#923=FACE_OUTER_BOUND('',#1337,.T.);
#924=FACE_OUTER_BOUND('',#1338,.T.);
#925=FACE_OUTER_BOUND('',#1339,.T.);
#926=FACE_OUTER_BOUND('',#1340,.T.);
#927=FACE_OUTER_BOUND('',#1341,.T.);
#928=FACE_OUTER_BOUND('',#1342,.T.);
#929=FACE_OUTER_BOUND('',#1343,.T.);
#930=FACE_OUTER_BOUND('',#1344,.T.);
#931=FACE_OUTER_BOUND('',#1345,.T.);
#932=FACE_OUTER_BOUND('',#1346,.T.);
#933=FACE_OUTER_BOUND('',#1347,.T.);
#934=FACE_OUTER_BOUND('',#1348,.T.);
#935=FACE_OUTER_BOUND('',#1349,.T.);
#936=FACE_OUTER_BOUND('',#1350,.T.);
#937=FACE_OUTER_BOUND('',#1351,.T.);
#938=FACE_OUTER_BOUND('',#1352,.T.);
#939=FACE_OUTER_BOUND('',#1353,.T.);
#940=FACE_OUTER_BOUND('',#1354,.T.);
#941=FACE_OUTER_BOUND('',#1355,.T.);
#942=FACE_OUTER_BOUND('',#1356,.T.);
#943=FACE_OUTER_BOUND('',#1357,.T.);
#944=FACE_OUTER_BOUND('',#1358,.T.);
#945=FACE_OUTER_BOUND('',#1359,.T.);
#946=FACE_OUTER_BOUND('',#1360,.T.);
#947=FACE_OUTER_BOUND('',#1361,.T.);
#948=FACE_OUTER_BOUND('',#1362,.T.);
#949=FACE_OUTER_BOUND('',#1363,.T.);
#950=FACE_OUTER_BOUND('',#1364,.T.);
#951=FACE_OUTER_BOUND('',#1365,.T.);
#952=FACE_OUTER_BOUND('',#1366,.T.);
#953=FACE_OUTER_BOUND('',#1367,.T.);
#954=FACE_OUTER_BOUND('',#1368,.T.);
#955=FACE_OUTER_BOUND('',#1369,.T.);
#956=FACE_OUTER_BOUND('',#1370,.T.);
#957=FACE_OUTER_BOUND('',#1371,.T.);
#958=FACE_OUTER_BOUND('',#1372,.T.);
#959=FACE_OUTER_BOUND('',#1373,.T.);
#960=FACE_OUTER_BOUND('',#1374,.T.);
#961=FACE_OUTER_BOUND('',#1375,.T.);
#962=FACE_OUTER_BOUND('',#1382,.T.);
#963=FACE_OUTER_BOUND('',#1383,.T.);
#1278=EDGE_LOOP('',(#4633,#4634,#4635,#4636,#4637,#4638,#4639,#4640));
#1279=EDGE_LOOP('',(#4641));
#1280=EDGE_LOOP('',(#4642));
#1281=EDGE_LOOP('',(#4643));
#1282=EDGE_LOOP('',(#4644,#4645,#4646,#4647));
#1283=EDGE_LOOP('',(#4648,#4649,#4650,#4651));
#1284=EDGE_LOOP('',(#4652,#4653,#4654,#4655));
#1285=EDGE_LOOP('',(#4656,#4657,#4658,#4659));
#1286=EDGE_LOOP('',(#4660,#4661,#4662,#4663));
#1287=EDGE_LOOP('',(#4664));
#1288=EDGE_LOOP('',(#4665));
#1289=EDGE_LOOP('',(#4666,#4667,#4668,#4669));
#1290=EDGE_LOOP('',(#4670));
#1291=EDGE_LOOP('',(#4671));
#1292=EDGE_LOOP('',(#4672,#4673,#4674,#4675));
#1293=EDGE_LOOP('',(#4676,#4677,#4678,#4679));
#1294=EDGE_LOOP('',(#4680,#4681,#4682,#4683));
#1295=EDGE_LOOP('',(#4684,#4685,#4686,#4687));
#1296=EDGE_LOOP('',(#4688,#4689,#4690,#4691));
#1297=EDGE_LOOP('',(#4692,#4693,#4694,#4695));
#1298=EDGE_LOOP('',(#4696,#4697,#4698,#4699));
#1299=EDGE_LOOP('',(#4700,#4701,#4702,#4703));
#1300=EDGE_LOOP('',(#4704,#4705,#4706,#4707));
#1301=EDGE_LOOP('',(#4708));
#1302=EDGE_LOOP('',(#4709));
#1303=EDGE_LOOP('',(#4710));
#1304=EDGE_LOOP('',(#4711));
#1305=EDGE_LOOP('',(#4712,#4713,#4714,#4715));
#1306=EDGE_LOOP('',(#4716,#4717,#4718,#4719));
#1307=EDGE_LOOP('',(#4720,#4721,#4722,#4723));
#1308=EDGE_LOOP('',(#4724,#4725,#4726,#4727));
#1309=EDGE_LOOP('',(#4728,#4729,#4730,#4731));
#1310=EDGE_LOOP('',(#4732,#4733,#4734,#4735,#4736,#4737));
#1311=EDGE_LOOP('',(#4738,#4739,#4740,#4741,#4742,#4743,#4744,#4745,#4746,
#4747));
#1312=EDGE_LOOP('',(#4748,#4749,#4750,#4751,#4752,#4753,#4754,#4755,#4756,
#4757));
#1313=EDGE_LOOP('',(#4758,#4759,#4760,#4761,#4762,#4763,#4764,#4765,#4766,
#4767));
#1314=EDGE_LOOP('',(#4768,#4769,#4770,#4771,#4772,#4773,#4774,#4775));
#1315=EDGE_LOOP('',(#4776,#4777,#4778,#4779,#4780,#4781,#4782,#4783,#4784,
#4785,#4786,#4787,#4788,#4789,#4790,#4791,#4792,#4793,#4794,#4795,#4796,
#4797,#4798,#4799,#4800,#4801,#4802,#4803,#4804,#4805,#4806,#4807,#4808,
#4809,#4810,#4811,#4812,#4813,#4814,#4815,#4816,#4817));
#1316=EDGE_LOOP('',(#4818,#4819,#4820,#4821,#4822,#4823));
#1317=EDGE_LOOP('',(#4824,#4825,#4826,#4827));
#1318=EDGE_LOOP('',(#4828,#4829,#4830,#4831));
#1319=EDGE_LOOP('',(#4832,#4833,#4834,#4835,#4836,#4837));
#1320=EDGE_LOOP('',(#4838,#4839,#4840,#4841));
#1321=EDGE_LOOP('',(#4842,#4843,#4844,#4845));
#1322=EDGE_LOOP('',(#4846,#4847,#4848,#4849));
#1323=EDGE_LOOP('',(#4850,#4851,#4852,#4853));
#1324=EDGE_LOOP('',(#4854,#4855,#4856,#4857));
#1325=EDGE_LOOP('',(#4858));
#1326=EDGE_LOOP('',(#4859));
#1327=EDGE_LOOP('',(#4860));
#1328=EDGE_LOOP('',(#4861,#4862,#4863,#4864));
#1329=EDGE_LOOP('',(#4865,#4866,#4867,#4868));
#1330=EDGE_LOOP('',(#4869,#4870,#4871,#4872));
#1331=EDGE_LOOP('',(#4873,#4874,#4875,#4876));
#1332=EDGE_LOOP('',(#4877,#4878,#4879,#4880,#4881,#4882,#4883,#4884,#4885,
#4886));
#1333=EDGE_LOOP('',(#4887,#4888,#4889,#4890));
#1334=EDGE_LOOP('',(#4891,#4892,#4893,#4894));
#1335=EDGE_LOOP('',(#4895,#4896,#4897,#4898));
#1336=EDGE_LOOP('',(#4899,#4900,#4901,#4902));
#1337=EDGE_LOOP('',(#4903,#4904,#4905,#4906));
#1338=EDGE_LOOP('',(#4907,#4908,#4909,#4910,#4911,#4912,#4913,#4914,#4915,
#4916));
#1339=EDGE_LOOP('',(#4917,#4918,#4919,#4920));
#1340=EDGE_LOOP('',(#4921,#4922,#4923,#4924,#4925,#4926));
#1341=EDGE_LOOP('',(#4927,#4928,#4929,#4930,#4931,#4932));
#1342=EDGE_LOOP('',(#4933,#4934,#4935,#4936));
#1343=EDGE_LOOP('',(#4937,#4938,#4939,#4940,#4941,#4942,#4943,#4944,#4945,
#4946));
#1344=EDGE_LOOP('',(#4947,#4948,#4949,#4950));
#1345=EDGE_LOOP('',(#4951,#4952,#4953,#4954));
#1346=EDGE_LOOP('',(#4955,#4956,#4957,#4958));
#1347=EDGE_LOOP('',(#4959,#4960,#4961,#4962));
#1348=EDGE_LOOP('',(#4963,#4964,#4965,#4966));
#1349=EDGE_LOOP('',(#4967,#4968,#4969));
#1350=EDGE_LOOP('',(#4970,#4971,#4972));
#1351=EDGE_LOOP('',(#4973,#4974,#4975));
#1352=EDGE_LOOP('',(#4976,#4977,#4978,#4979));
#1353=EDGE_LOOP('',(#4980,#4981,#4982,#4983));
#1354=EDGE_LOOP('',(#4984,#4985,#4986));
#1355=EDGE_LOOP('',(#4987,#4988,#4989,#4990));
#1356=EDGE_LOOP('',(#4991,#4992,#4993,#4994));
#1357=EDGE_LOOP('',(#4995,#4996,#4997,#4998));
#1358=EDGE_LOOP('',(#4999,#5000,#5001,#5002));
#1359=EDGE_LOOP('',(#5003,#5004,#5005,#5006));
#1360=EDGE_LOOP('',(#5007,#5008,#5009,#5010));
#1361=EDGE_LOOP('',(#5011,#5012,#5013));
#1362=EDGE_LOOP('',(#5014,#5015,#5016));
#1363=EDGE_LOOP('',(#5017,#5018,#5019));
#1364=EDGE_LOOP('',(#5020,#5021,#5022,#5023));
#1365=EDGE_LOOP('',(#5024,#5025,#5026,#5027));
#1366=EDGE_LOOP('',(#5028,#5029,#5030));
#1367=EDGE_LOOP('',(#5031,#5032,#5033,#5034));
#1368=EDGE_LOOP('',(#5035,#5036,#5037,#5038));
#1369=EDGE_LOOP('',(#5039,#5040,#5041,#5042));
#1370=EDGE_LOOP('',(#5043,#5044,#5045,#5046));
#1371=EDGE_LOOP('',(#5047,#5048,#5049,#5050));
#1372=EDGE_LOOP('',(#5051,#5052,#5053,#5054));
#1373=EDGE_LOOP('',(#5055,#5056,#5057,#5058));
#1374=EDGE_LOOP('',(#5059,#5060,#5061,#5062,#5063,#5064,#5065,#5066));
#1375=EDGE_LOOP('',(#5067,#5068,#5069,#5070));
#1376=EDGE_LOOP('',(#5071));
#1377=EDGE_LOOP('',(#5072));
#1378=EDGE_LOOP('',(#5073));
#1379=EDGE_LOOP('',(#5074));
#1380=EDGE_LOOP('',(#5075));
#1381=EDGE_LOOP('',(#5076));
#1382=EDGE_LOOP('',(#5077,#5078,#5079,#5080));
#1383=EDGE_LOOP('',(#5081,#5082,#5083,#5084));
#1773=LINE('',#9202,#2222);
#1774=LINE('',#9234,#2223);
#1775=LINE('',#9269,#2224);
#1776=LINE('',#9274,#2225);
#1777=LINE('',#9278,#2226);
#1778=LINE('',#9283,#2227);
#1779=LINE('',#9289,#2228);
#1780=LINE('',#9298,#2229);
#1781=LINE('',#9305,#2230);
#1782=LINE('',#9309,#2231);
#1783=LINE('',#9314,#2232);
#1784=LINE('',#9316,#2233);
#1785=LINE('',#9318,#2234);
#1786=LINE('',#9319,#2235);
#1787=LINE('',#9323,#2236);
#1788=LINE('',#9325,#2237);
#1789=LINE('',#9327,#2238);
#1790=LINE('',#9328,#2239);
#1791=LINE('',#9332,#2240);
#1792=LINE('',#9334,#2241);
#1793=LINE('',#9336,#2242);
#1794=LINE('',#9337,#2243);
#1795=LINE('',#9341,#2244);
#1796=LINE('',#9343,#2245);
#1797=LINE('',#9345,#2246);
#1798=LINE('',#9346,#2247);
#1799=LINE('',#9350,#2248);
#1800=LINE('',#9352,#2249);
#1801=LINE('',#9354,#2250);
#1802=LINE('',#9355,#2251);
#1803=LINE('',#9359,#2252);
#1804=LINE('',#9361,#2253);
#1805=LINE('',#9363,#2254);
#1806=LINE('',#9364,#2255);
#1807=LINE('',#9368,#2256);
#1808=LINE('',#9370,#2257);
#1809=LINE('',#9372,#2258);
#1810=LINE('',#9373,#2259);
#1811=LINE('',#9381,#2260);
#1812=LINE('',#9382,#2261);
#1813=LINE('',#9384,#2262);
#1814=LINE('',#9385,#2263);
#1815=LINE('',#9387,#2264);
#1816=LINE('',#9388,#2265);
#1817=LINE('',#9391,#2266);
#1818=LINE('',#9393,#2267);
#1819=LINE('',#9394,#2268);
#1820=LINE('',#9397,#2269);
#1821=LINE('',#9399,#2270);
#1822=LINE('',#9400,#2271);
#1823=LINE('',#9404,#2272);
#1824=LINE('',#9442,#2273);
#1825=LINE('',#9480,#2274);
#1826=LINE('',#9518,#2275);
#1827=LINE('',#9555,#2276);
#1828=LINE('',#9558,#2277);
#1829=LINE('',#9596,#2278);
#1830=LINE('',#9633,#2279);
#1831=LINE('',#9636,#2280);
#1832=LINE('',#9708,#2281);
#1833=LINE('',#9711,#2282);
#1834=LINE('',#9718,#2283);
#1835=LINE('',#9724,#2284);
#1836=LINE('',#9735,#2285);
#1837=LINE('',#9747,#2286);
#1838=LINE('',#9753,#2287);
#1839=LINE('',#9788,#2288);
#1840=LINE('',#9877,#2289);
#1841=LINE('',#9965,#2290);
#1842=LINE('',#10000,#2291);
#1843=LINE('',#10006,#2292);
#1844=LINE('',#10018,#2293);
#1845=LINE('',#10061,#2294);
#1846=LINE('',#10102,#2295);
#1847=LINE('',#10106,#2296);
#1848=LINE('',#10108,#2297);
#1849=LINE('',#10154,#2298);
#1850=LINE('',#10289,#2299);
#1851=LINE('',#10393,#2300);
#1852=LINE('',#10707,#2301);
#1853=LINE('',#10796,#2302);
#1854=LINE('',#10884,#2303);
#1855=LINE('',#11004,#2304);
#1856=LINE('',#11005,#2305);
#1857=LINE('',#11042,#2306);
#1858=LINE('',#11043,#2307);
#2222=VECTOR('',#7758,1.);
#2223=VECTOR('',#7759,1.);
#2224=VECTOR('',#7770,0.15);
#2225=VECTOR('',#7777,0.15);
#2226=VECTOR('',#7782,0.15);
#2227=VECTOR('',#7787,0.15);
#2228=VECTOR('',#7794,0.3);
#2229=VECTOR('',#7805,0.3);
#2230=VECTOR('',#7814,0.17);
#2231=VECTOR('',#7819,0.17);
#2232=VECTOR('',#7824,1.);
#2233=VECTOR('',#7825,1.);
#2234=VECTOR('',#7826,1.);
#2235=VECTOR('',#7827,1.);
#2236=VECTOR('',#7830,1.);
#2237=VECTOR('',#7831,1.);
#2238=VECTOR('',#7832,1.);
#2239=VECTOR('',#7833,1.);
#2240=VECTOR('',#7836,1.);
#2241=VECTOR('',#7837,1.);
#2242=VECTOR('',#7838,1.);
#2243=VECTOR('',#7839,1.);
#2244=VECTOR('',#7842,1.);
#2245=VECTOR('',#7843,1.);
#2246=VECTOR('',#7844,1.);
#2247=VECTOR('',#7845,1.);
#2248=VECTOR('',#7848,1.);
#2249=VECTOR('',#7849,1.);
#2250=VECTOR('',#7850,1.);
#2251=VECTOR('',#7851,1.);
#2252=VECTOR('',#7854,1.);
#2253=VECTOR('',#7855,1.);
#2254=VECTOR('',#7856,1.);
#2255=VECTOR('',#7857,1.);
#2256=VECTOR('',#7860,1.);
#2257=VECTOR('',#7861,1.);
#2258=VECTOR('',#7862,1.);
#2259=VECTOR('',#7863,1.);
#2260=VECTOR('',#7874,1.);
#2261=VECTOR('',#7875,1.);
#2262=VECTOR('',#7878,1.);
#2263=VECTOR('',#7879,1.);
#2264=VECTOR('',#7882,1.);
#2265=VECTOR('',#7883,1.);
#2266=VECTOR('',#7886,1.);
#2267=VECTOR('',#7887,1.);
#2268=VECTOR('',#7888,1.);
#2269=VECTOR('',#7891,1.);
#2270=VECTOR('',#7892,1.);
#2271=VECTOR('',#7893,1.);
#2272=VECTOR('',#7896,1.);
#2273=VECTOR('',#7897,1.);
#2274=VECTOR('',#7900,1.);
#2275=VECTOR('',#7901,1.);
#2276=VECTOR('',#7902,1.);
#2277=VECTOR('',#7905,1.);
#2278=VECTOR('',#7906,1.);
#2279=VECTOR('',#7907,1.);
#2280=VECTOR('',#7910,1.);
#2281=VECTOR('',#7911,1.);
#2282=VECTOR('',#7914,1.);
#2283=VECTOR('',#7915,1.);
#2284=VECTOR('',#7916,1.);
#2285=VECTOR('',#7919,1.);
#2286=VECTOR('',#7920,1.);
#2287=VECTOR('',#7921,1.);
#2288=VECTOR('',#7922,1.);
#2289=VECTOR('',#7923,1.);
#2290=VECTOR('',#7924,1.);
#2291=VECTOR('',#7925,1.);
#2292=VECTOR('',#7926,1.);
#2293=VECTOR('',#7927,1.);
#2294=VECTOR('',#7928,1.);
#2295=VECTOR('',#7929,1.);
#2296=VECTOR('',#7934,0.4);
#2297=VECTOR('',#7937,0.4);
#2298=VECTOR('',#7940,1.);
#2299=VECTOR('',#7947,1.);
#2300=VECTOR('',#7950,1.);
#2301=VECTOR('',#7957,1.);
#2302=VECTOR('',#7962,1.);
#2303=VECTOR('',#7995,1.);
#2304=VECTOR('',#8024,1.);
#2305=VECTOR('',#8025,1.);
#2306=VECTOR('',#8036,1.);
#2307=VECTOR('',#8037,1.);
#2586=CIRCLE('',#7043,0.15);
#2587=CIRCLE('',#7044,0.15);
#2588=CIRCLE('',#7045,0.4);
#2589=CIRCLE('',#7047,0.15);
#2590=CIRCLE('',#7048,0.15);
#2591=CIRCLE('',#7050,0.15);
#2592=CIRCLE('',#7052,0.15);
#2593=CIRCLE('',#7054,0.15);
#2594=CIRCLE('',#7055,0.15);
#2595=CIRCLE('',#7057,0.3);
#2596=CIRCLE('',#7058,0.3);
#2597=CIRCLE('',#7060,0.17);
#2598=CIRCLE('',#7062,0.3);
#2599=CIRCLE('',#7063,0.3);
#2600=CIRCLE('',#7065,0.17);
#2601=CIRCLE('',#7067,0.17);
#2602=CIRCLE('',#7069,0.17);
#2603=CIRCLE('',#7078,0.4);
#2604=CIRCLE('',#7080,0.4);
#2605=CIRCLE('',#7093,0.4);
#2606=CIRCLE('',#7096,0.1);
#2607=CIRCLE('',#7103,0.0999999999999999);
#2608=CIRCLE('',#7105,0.0999999999999999);
#2609=CIRCLE('',#7107,0.0999999999999999);
#2610=CIRCLE('',#7108,0.1);
#2611=CIRCLE('',#7110,0.0999999999999998);
#2612=CIRCLE('',#7111,0.0999999999999998);
#2613=CIRCLE('',#7112,0.0999999999999997);
#2614=CIRCLE('',#7114,0.0999999999999998);
#2615=CIRCLE('',#7115,0.0999999999999998);
#2616=CIRCLE('',#7118,0.0999999999999999);
#2617=CIRCLE('',#7119,0.1);
#2618=CIRCLE('',#7123,0.3);
#2619=CIRCLE('',#7124,0.3);
#2620=CIRCLE('',#7125,0.3);
#2621=CIRCLE('',#7127,0.3);
#2622=CIRCLE('',#7128,0.3);
#2623=CIRCLE('',#7129,0.3);
#2624=CIRCLE('',#7131,0.3);
#2625=CIRCLE('',#7132,0.3);
#2626=CIRCLE('',#7133,0.3);
#2627=CIRCLE('',#7136,0.3);
#2628=CIRCLE('',#7137,0.3);
#2629=CIRCLE('',#7138,0.3);
#2812=VERTEX_POINT('',#9195);
#2813=VERTEX_POINT('',#9196);
#2814=VERTEX_POINT('',#9201);
#2815=VERTEX_POINT('',#9203);
#2816=VERTEX_POINT('',#9208);
#2817=VERTEX_POINT('',#9228);
#2818=VERTEX_POINT('',#9233);
#2819=VERTEX_POINT('',#9235);
#2820=VERTEX_POINT('',#9259);
#2821=VERTEX_POINT('',#9261);
#2822=VERTEX_POINT('',#9263);
#2823=VERTEX_POINT('',#9266);
#2824=VERTEX_POINT('',#9268);
#2825=VERTEX_POINT('',#9272);
#2826=VERTEX_POINT('',#9276);
#2827=VERTEX_POINT('',#9280);
#2828=VERTEX_POINT('',#9282);
#2829=VERTEX_POINT('',#9286);
#2830=VERTEX_POINT('',#9288);
#2831=VERTEX_POINT('',#9292);
#2832=VERTEX_POINT('',#9295);
#2833=VERTEX_POINT('',#9297);
#2834=VERTEX_POINT('',#9301);
#2835=VERTEX_POINT('',#9304);
#2836=VERTEX_POINT('',#9308);
#2837=VERTEX_POINT('',#9312);
#2838=VERTEX_POINT('',#9313);
#2839=VERTEX_POINT('',#9315);
#2840=VERTEX_POINT('',#9317);
#2841=VERTEX_POINT('',#9321);
#2842=VERTEX_POINT('',#9322);
#2843=VERTEX_POINT('',#9324);
#2844=VERTEX_POINT('',#9326);
#2845=VERTEX_POINT('',#9330);
#2846=VERTEX_POINT('',#9331);
#2847=VERTEX_POINT('',#9333);
#2848=VERTEX_POINT('',#9335);
#2849=VERTEX_POINT('',#9339);
#2850=VERTEX_POINT('',#9340);
#2851=VERTEX_POINT('',#9342);
#2852=VERTEX_POINT('',#9344);
#2853=VERTEX_POINT('',#9348);
#2854=VERTEX_POINT('',#9349);
#2855=VERTEX_POINT('',#9351);
#2856=VERTEX_POINT('',#9353);
#2857=VERTEX_POINT('',#9357);
#2858=VERTEX_POINT('',#9358);
#2859=VERTEX_POINT('',#9360);
#2860=VERTEX_POINT('',#9362);
#2861=VERTEX_POINT('',#9366);
#2862=VERTEX_POINT('',#9367);
#2863=VERTEX_POINT('',#9369);
#2864=VERTEX_POINT('',#9371);
#2865=VERTEX_POINT('',#9375);
#2866=VERTEX_POINT('',#9378);
#2867=VERTEX_POINT('',#9390);
#2868=VERTEX_POINT('',#9392);
#2869=VERTEX_POINT('',#9396);
#2870=VERTEX_POINT('',#9398);
#2871=VERTEX_POINT('',#9402);
#2872=VERTEX_POINT('',#9403);
#2873=VERTEX_POINT('',#9405);
#2874=VERTEX_POINT('',#9412);
#2875=VERTEX_POINT('',#9441);
#2876=VERTEX_POINT('',#9443);
#2877=VERTEX_POINT('',#9479);
#2878=VERTEX_POINT('',#9481);
#2879=VERTEX_POINT('',#9488);
#2880=VERTEX_POINT('',#9517);
#2881=VERTEX_POINT('',#9519);
#2882=VERTEX_POINT('',#9548);
#2883=VERTEX_POINT('',#9557);
#2884=VERTEX_POINT('',#9559);
#2885=VERTEX_POINT('',#9566);
#2886=VERTEX_POINT('',#9595);
#2887=VERTEX_POINT('',#9597);
#2888=VERTEX_POINT('',#9626);
#2889=VERTEX_POINT('',#9635);
#2890=VERTEX_POINT('',#9637);
#2891=VERTEX_POINT('',#9672);
#2892=VERTEX_POINT('',#9701);
#2893=VERTEX_POINT('',#9710);
#2894=VERTEX_POINT('',#9712);
#2895=VERTEX_POINT('',#9717);
#2896=VERTEX_POINT('',#9719);
#2897=VERTEX_POINT('',#9734);
#2898=VERTEX_POINT('',#9746);
#2899=VERTEX_POINT('',#9752);
#2900=VERTEX_POINT('',#9754);
#2901=VERTEX_POINT('',#9787);
#2902=VERTEX_POINT('',#9789);
#2903=VERTEX_POINT('',#9827);
#2904=VERTEX_POINT('',#9832);
#2905=VERTEX_POINT('',#9876);
#2906=VERTEX_POINT('',#9878);
#2907=VERTEX_POINT('',#9922);
#2908=VERTEX_POINT('',#9927);
#2909=VERTEX_POINT('',#9966);
#2910=VERTEX_POINT('',#9995);
#2911=VERTEX_POINT('',#10001);
#2912=VERTEX_POINT('',#10007);
#2913=VERTEX_POINT('',#10019);
#2914=VERTEX_POINT('',#10020);
#2915=VERTEX_POINT('',#10025);
#2916=VERTEX_POINT('',#10060);
#2917=VERTEX_POINT('',#10062);
#2918=VERTEX_POINT('',#10097);
#2919=VERTEX_POINT('',#10104);
#2920=VERTEX_POINT('',#10110);
#2921=VERTEX_POINT('',#10117);
#2922=VERTEX_POINT('',#10124);
#2923=VERTEX_POINT('',#10153);
#2924=VERTEX_POINT('',#10219);
#2925=VERTEX_POINT('',#10272);
#2926=VERTEX_POINT('',#10284);
#2927=VERTEX_POINT('',#10346);
#2928=VERTEX_POINT('',#10356);
#2929=VERTEX_POINT('',#10363);
#2930=VERTEX_POINT('',#10392);
#2931=VERTEX_POINT('',#10394);
#2932=VERTEX_POINT('',#10519);
#2933=VERTEX_POINT('',#10554);
#2934=VERTEX_POINT('',#10670);
#2935=VERTEX_POINT('',#10677);
#2936=VERTEX_POINT('',#10706);
#2937=VERTEX_POINT('',#10708);
#2938=VERTEX_POINT('',#10759);
#2939=VERTEX_POINT('',#10788);
#2940=VERTEX_POINT('',#10795);
#2941=VERTEX_POINT('',#10817);
#2942=VERTEX_POINT('',#10852);
#2943=VERTEX_POINT('',#10880);
#2944=VERTEX_POINT('',#10983);
#2945=VERTEX_POINT('',#10984);
#2946=VERTEX_POINT('',#10986);
#2947=VERTEX_POINT('',#10990);
#2948=VERTEX_POINT('',#10991);
#2949=VERTEX_POINT('',#10993);
#2950=VERTEX_POINT('',#10997);
#2951=VERTEX_POINT('',#10998);
#2952=VERTEX_POINT('',#11000);
#2953=VERTEX_POINT('',#11035);
#2954=VERTEX_POINT('',#11036);
#2955=VERTEX_POINT('',#11038);
#3501=EDGE_CURVE('',#2812,#2813,#172,.T.);
#3502=EDGE_CURVE('',#2813,#2814,#1773,.T.);
#3503=EDGE_CURVE('',#2814,#2815,#173,.T.);
#3504=EDGE_CURVE('',#2816,#2815,#174,.T.);
#3505=EDGE_CURVE('',#2816,#2817,#175,.T.);
#3506=EDGE_CURVE('',#2817,#2818,#1774,.T.);
#3507=EDGE_CURVE('',#2818,#2819,#176,.T.);
#3508=EDGE_CURVE('',#2812,#2819,#177,.T.);
#3509=EDGE_CURVE('',#2820,#2820,#2586,.T.);
#3510=EDGE_CURVE('',#2821,#2821,#2587,.T.);
#3511=EDGE_CURVE('',#2822,#2822,#2588,.T.);
#3512=EDGE_CURVE('',#2823,#2823,#2589,.T.);
#3513=EDGE_CURVE('',#2823,#2824,#1775,.T.);
#3514=EDGE_CURVE('',#2824,#2824,#2590,.T.);
#3515=EDGE_CURVE('',#2825,#2825,#2591,.T.);
#3516=EDGE_CURVE('',#2825,#2821,#1776,.T.);
#3517=EDGE_CURVE('',#2826,#2826,#2592,.T.);
#3518=EDGE_CURVE('',#2826,#2820,#1777,.T.);
#3519=EDGE_CURVE('',#2827,#2827,#2593,.T.);
#3520=EDGE_CURVE('',#2827,#2828,#1778,.T.);
#3521=EDGE_CURVE('',#2828,#2828,#2594,.T.);
#3522=EDGE_CURVE('',#2829,#2829,#2595,.T.);
#3523=EDGE_CURVE('',#2829,#2830,#1779,.T.);
#3524=EDGE_CURVE('',#2830,#2830,#2596,.T.);
#3525=EDGE_CURVE('',#2831,#2831,#2597,.T.);
#3526=EDGE_CURVE('',#2832,#2832,#2598,.T.);
#3527=EDGE_CURVE('',#2832,#2833,#1780,.T.);
#3528=EDGE_CURVE('',#2833,#2833,#2599,.T.);
#3529=EDGE_CURVE('',#2834,#2834,#2600,.T.);
#3530=EDGE_CURVE('',#2831,#2835,#1781,.T.);
#3531=EDGE_CURVE('',#2835,#2835,#2601,.T.);
#3532=EDGE_CURVE('',#2834,#2836,#1782,.T.);
#3533=EDGE_CURVE('',#2836,#2836,#2602,.T.);
#3534=EDGE_CURVE('',#2837,#2838,#1783,.T.);
#3535=EDGE_CURVE('',#2839,#2837,#1784,.T.);
#3536=EDGE_CURVE('',#2840,#2839,#1785,.T.);
#3537=EDGE_CURVE('',#2840,#2838,#1786,.T.);
#3538=EDGE_CURVE('',#2841,#2842,#1787,.T.);
#3539=EDGE_CURVE('',#2841,#2843,#1788,.T.);
#3540=EDGE_CURVE('',#2844,#2843,#1789,.T.);
#3541=EDGE_CURVE('',#2842,#2844,#1790,.T.);
#3542=EDGE_CURVE('',#2845,#2846,#1791,.T.);
#3543=EDGE_CURVE('',#2845,#2847,#1792,.T.);
#3544=EDGE_CURVE('',#2848,#2847,#1793,.T.);
#3545=EDGE_CURVE('',#2846,#2848,#1794,.T.);
#3546=EDGE_CURVE('',#2849,#2850,#1795,.T.);
#3547=EDGE_CURVE('',#2849,#2851,#1796,.T.);
#3548=EDGE_CURVE('',#2852,#2851,#1797,.T.);
#3549=EDGE_CURVE('',#2850,#2852,#1798,.T.);
#3550=EDGE_CURVE('',#2853,#2854,#1799,.T.);
#3551=EDGE_CURVE('',#2853,#2855,#1800,.T.);
#3552=EDGE_CURVE('',#2856,#2855,#1801,.T.);
#3553=EDGE_CURVE('',#2854,#2856,#1802,.T.);
#3554=EDGE_CURVE('',#2857,#2858,#1803,.T.);
#3555=EDGE_CURVE('',#2859,#2857,#1804,.T.);
#3556=EDGE_CURVE('',#2860,#2859,#1805,.T.);
#3557=EDGE_CURVE('',#2860,#2858,#1806,.T.);
#3558=EDGE_CURVE('',#2861,#2862,#1807,.T.);
#3559=EDGE_CURVE('',#2863,#2861,#1808,.T.);
#3560=EDGE_CURVE('',#2864,#2863,#1809,.T.);
#3561=EDGE_CURVE('',#2864,#2862,#1810,.T.);
#3562=EDGE_CURVE('',#2865,#2865,#2603,.T.);
#3563=EDGE_CURVE('',#2866,#2866,#2604,.T.);
#3564=EDGE_CURVE('',#2838,#2853,#1811,.T.);
#3565=EDGE_CURVE('',#2855,#2840,#1812,.T.);
#3566=EDGE_CURVE('',#2858,#2841,#1813,.T.);
#3567=EDGE_CURVE('',#2843,#2860,#1814,.T.);
#3568=EDGE_CURVE('',#2862,#2845,#1815,.T.);
#3569=EDGE_CURVE('',#2847,#2864,#1816,.T.);
#3570=EDGE_CURVE('',#2867,#2849,#1817,.T.);
#3571=EDGE_CURVE('',#2868,#2867,#1818,.T.);
#3572=EDGE_CURVE('',#2851,#2868,#1819,.T.);
#3573=EDGE_CURVE('',#2869,#2867,#1820,.T.);
#3574=EDGE_CURVE('',#2870,#2869,#1821,.T.);
#3575=EDGE_CURVE('',#2868,#2870,#1822,.T.);
#3576=EDGE_CURVE('',#2871,#2872,#1823,.T.);
#3577=EDGE_CURVE('',#2873,#2872,#178,.T.);
#3578=EDGE_CURVE('',#2874,#2873,#179,.T.);
#3579=EDGE_CURVE('',#2875,#2874,#1824,.T.);
#3580=EDGE_CURVE('',#2876,#2875,#180,.T.);
#3581=EDGE_CURVE('',#2871,#2876,#181,.T.);
#3582=EDGE_CURVE('',#2870,#2877,#1825,.T.);
#3583=EDGE_CURVE('',#2878,#2877,#182,.T.);
#3584=EDGE_CURVE('',#2879,#2878,#183,.T.);
#3585=EDGE_CURVE('',#2880,#2879,#1826,.T.);
#3586=EDGE_CURVE('',#2881,#2880,#184,.T.);
#3587=EDGE_CURVE('',#2882,#2881,#185,.T.);
#3588=EDGE_CURVE('',#2882,#2852,#1827,.T.);
#3589=EDGE_CURVE('',#2863,#2883,#1828,.T.);
#3590=EDGE_CURVE('',#2884,#2883,#186,.T.);
#3591=EDGE_CURVE('',#2885,#2884,#187,.T.);
#3592=EDGE_CURVE('',#2886,#2885,#1829,.T.);
#3593=EDGE_CURVE('',#2887,#2886,#188,.T.);
#3594=EDGE_CURVE('',#2888,#2887,#189,.T.);
#3595=EDGE_CURVE('',#2888,#2848,#1830,.T.);
#3596=EDGE_CURVE('',#2859,#2889,#1831,.T.);
#3597=EDGE_CURVE('',#2890,#2889,#190,.T.);
#3598=EDGE_CURVE('',#2818,#2890,#191,.T.);
#3599=EDGE_CURVE('',#2891,#2817,#192,.T.);
#3600=EDGE_CURVE('',#2892,#2891,#193,.T.);
#3601=EDGE_CURVE('',#2892,#2844,#1832,.T.);
#3602=EDGE_CURVE('',#2893,#2854,#1833,.T.);
#3603=EDGE_CURVE('',#2893,#2894,#194,.T.);
#3604=EDGE_CURVE('',#2894,#2895,#1834,.T.);
#3605=EDGE_CURVE('',#2895,#2896,#195,.T.);
#3606=EDGE_CURVE('',#2837,#2896,#1835,.T.);
#3607=EDGE_CURVE('',#2882,#2872,#196,.T.);
#3608=EDGE_CURVE('',#2871,#2877,#197,.T.);
#3609=EDGE_CURVE('',#2897,#2869,#1836,.T.);
#3610=EDGE_CURVE('',#2897,#2883,#198,.T.);
#3611=EDGE_CURVE('',#2898,#2861,#1837,.T.);
#3612=EDGE_CURVE('',#2898,#2889,#199,.T.);
#3613=EDGE_CURVE('',#2899,#2857,#1838,.T.);
#3614=EDGE_CURVE('',#2899,#2900,#200,.T.);
#3615=EDGE_CURVE('',#2900,#2893,#201,.T.);
#3616=EDGE_CURVE('',#2856,#2901,#1839,.T.);
#3617=EDGE_CURVE('',#2902,#2901,#202,.T.);
#3618=EDGE_CURVE('',#2902,#2903,#203,.T.);
#3619=EDGE_CURVE('',#2904,#2903,#204,.T.);
#3620=EDGE_CURVE('',#2904,#2905,#1840,.T.);
#3621=EDGE_CURVE('',#2906,#2905,#205,.T.);
#3622=EDGE_CURVE('',#2906,#2907,#206,.T.);
#3623=EDGE_CURVE('',#2908,#2907,#207,.T.);
#3624=EDGE_CURVE('',#2908,#2839,#1841,.T.);
#3625=EDGE_CURVE('',#2896,#2909,#208,.T.);
#3626=EDGE_CURVE('',#2909,#2910,#209,.T.);
#3627=EDGE_CURVE('',#2842,#2910,#1842,.T.);
#3628=EDGE_CURVE('',#2892,#2911,#210,.T.);
#3629=EDGE_CURVE('',#2846,#2911,#1843,.T.);
#3630=EDGE_CURVE('',#2888,#2912,#211,.T.);
#3631=EDGE_CURVE('',#2850,#2912,#1844,.T.);
#3632=EDGE_CURVE('',#2913,#2914,#212,.T.);
#3633=EDGE_CURVE('',#2914,#2915,#213,.T.);
#3634=EDGE_CURVE('',#2915,#2916,#1845,.T.);
#3635=EDGE_CURVE('',#2916,#2917,#214,.T.);
#3636=EDGE_CURVE('',#2917,#2918,#215,.T.);
#3637=EDGE_CURVE('',#2913,#2918,#1846,.T.);
#3638=EDGE_CURVE('',#2919,#2919,#2605,.T.);
#3639=EDGE_CURVE('',#2919,#2866,#1847,.T.);
#3640=EDGE_CURVE('',#2822,#2865,#1848,.T.);
#3641=EDGE_CURVE('',#2913,#2920,#216,.T.);
#3642=EDGE_CURVE('',#2921,#2918,#217,.T.);
#3643=EDGE_CURVE('',#2922,#2921,#218,.T.);
#3644=EDGE_CURVE('',#2923,#2922,#1849,.T.);
#3645=EDGE_CURVE('',#2920,#2923,#219,.T.);
#3646=EDGE_CURVE('',#2881,#2873,#220,.T.);
#3647=EDGE_CURVE('',#2920,#2924,#221,.T.);
#3648=EDGE_CURVE('',#2924,#2914,#222,.T.);
#3649=EDGE_CURVE('',#2874,#2880,#223,.T.);
#3650=EDGE_CURVE('',#2925,#2923,#224,.T.);
#3651=EDGE_CURVE('',#2924,#2925,#2606,.F.);
#3652=EDGE_CURVE('',#2879,#2875,#225,.T.);
#3653=EDGE_CURVE('',#2922,#2926,#226,.T.);
#3654=EDGE_CURVE('',#2926,#2925,#1850,.T.);
#3655=EDGE_CURVE('',#2876,#2878,#227,.T.);
#3656=EDGE_CURVE('',#2917,#2927,#228,.T.);
#3657=EDGE_CURVE('',#2927,#2921,#229,.T.);
#3658=EDGE_CURVE('',#2928,#2912,#230,.T.);
#3659=EDGE_CURVE('',#2929,#2928,#231,.T.);
#3660=EDGE_CURVE('',#2930,#2929,#1851,.T.);
#3661=EDGE_CURVE('',#2931,#2930,#232,.T.);
#3662=EDGE_CURVE('',#2897,#2931,#233,.T.);
#3663=EDGE_CURVE('',#2887,#2928,#234,.T.);
#3664=EDGE_CURVE('',#2929,#2886,#235,.T.);
#3665=EDGE_CURVE('',#2885,#2930,#236,.T.);
#3666=EDGE_CURVE('',#2931,#2884,#237,.T.);
#3667=EDGE_CURVE('',#2932,#2911,#238,.T.);
#3668=EDGE_CURVE('',#2814,#2932,#239,.T.);
#3669=EDGE_CURVE('',#2933,#2813,#240,.T.);
#3670=EDGE_CURVE('',#2898,#2933,#241,.T.);
#3671=EDGE_CURVE('',#2891,#2932,#242,.T.);
#3672=EDGE_CURVE('',#2933,#2890,#243,.T.);
#3673=EDGE_CURVE('',#2934,#2910,#244,.T.);
#3674=EDGE_CURVE('',#2935,#2934,#245,.T.);
#3675=EDGE_CURVE('',#2936,#2935,#1852,.T.);
#3676=EDGE_CURVE('',#2937,#2936,#246,.T.);
#3677=EDGE_CURVE('',#2899,#2937,#247,.T.);
#3678=EDGE_CURVE('',#2909,#2938,#248,.T.);
#3679=EDGE_CURVE('',#2938,#2934,#249,.T.);
#3680=EDGE_CURVE('',#2939,#2938,#2607,.F.);
#3681=EDGE_CURVE('',#2935,#2939,#250,.T.);
#3682=EDGE_CURVE('',#2939,#2940,#1853,.T.);
#3683=EDGE_CURVE('',#2940,#2936,#251,.T.);
#3684=EDGE_CURVE('',#2937,#2941,#252,.T.);
#3685=EDGE_CURVE('',#2941,#2900,#253,.T.);
#3686=EDGE_CURVE('',#2941,#2940,#2608,.F.);
#3687=EDGE_CURVE('',#2940,#2894,#2609,.F.);
#3688=EDGE_CURVE('',#2894,#2941,#2610,.F.);
#3689=EDGE_CURVE('',#2926,#2927,#2611,.F.);
#3690=EDGE_CURVE('',#2927,#2942,#2612,.F.);
#3691=EDGE_CURVE('',#2942,#2926,#2613,.F.);
#3692=EDGE_CURVE('',#2938,#2895,#2614,.F.);
#3693=EDGE_CURVE('',#2895,#2939,#2615,.F.);
#3694=EDGE_CURVE('',#2943,#2924,#2616,.F.);
#3695=EDGE_CURVE('',#2925,#2943,#2617,.F.);
#3696=EDGE_CURVE('',#2943,#2942,#1854,.T.);
#3697=EDGE_CURVE('',#2915,#2943,#254,.T.);
#3698=EDGE_CURVE('',#2942,#2916,#255,.T.);
#3699=EDGE_CURVE('',#2944,#2945,#2618,.F.);
#3700=EDGE_CURVE('',#2946,#2944,#2619,.F.);
#3701=EDGE_CURVE('',#2945,#2946,#2620,.F.);
#3702=EDGE_CURVE('',#2947,#2948,#2621,.F.);
#3703=EDGE_CURVE('',#2949,#2947,#2622,.F.);
#3704=EDGE_CURVE('',#2948,#2949,#2623,.F.);
#3705=EDGE_CURVE('',#2950,#2951,#2624,.F.);
#3706=EDGE_CURVE('',#2952,#2950,#2625,.F.);
#3707=EDGE_CURVE('',#2951,#2952,#2626,.F.);
#3708=EDGE_CURVE('',#2945,#2952,#1855,.T.);
#3709=EDGE_CURVE('',#2950,#2944,#1856,.T.);
#3710=EDGE_CURVE('',#2907,#2951,#256,.T.);
#3711=EDGE_CURVE('',#2952,#2908,#257,.T.);
#3712=EDGE_CURVE('',#2953,#2954,#2627,.F.);
#3713=EDGE_CURVE('',#2955,#2953,#2628,.F.);
#3714=EDGE_CURVE('',#2954,#2955,#2629,.F.);
#3715=EDGE_CURVE('',#2953,#2949,#1857,.T.);
#3716=EDGE_CURVE('',#2947,#2955,#1858,.T.);
#3717=EDGE_CURVE('',#2951,#2954,#258,.T.);
#3718=EDGE_CURVE('',#2955,#2950,#259,.T.);
#3719=EDGE_CURVE('',#2905,#2953,#260,.T.);
#3720=EDGE_CURVE('',#2954,#2906,#261,.T.);
#3721=EDGE_CURVE('',#2903,#2948,#262,.T.);
#3722=EDGE_CURVE('',#2949,#2904,#263,.T.);
#3723=EDGE_CURVE('',#2948,#2946,#264,.T.);
#3724=EDGE_CURVE('',#2944,#2947,#265,.T.);
#3725=EDGE_CURVE('',#2901,#2945,#266,.T.);
#3726=EDGE_CURVE('',#2946,#2902,#267,.T.);
#4633=ORIENTED_EDGE('',*,*,#3501,.T.);
#4634=ORIENTED_EDGE('',*,*,#3502,.T.);
#4635=ORIENTED_EDGE('',*,*,#3503,.T.);
#4636=ORIENTED_EDGE('',*,*,#3504,.F.);
#4637=ORIENTED_EDGE('',*,*,#3505,.T.);
#4638=ORIENTED_EDGE('',*,*,#3506,.T.);
#4639=ORIENTED_EDGE('',*,*,#3507,.T.);
#4640=ORIENTED_EDGE('',*,*,#3508,.F.);
#4641=ORIENTED_EDGE('',*,*,#3509,.T.);
#4642=ORIENTED_EDGE('',*,*,#3510,.T.);
#4643=ORIENTED_EDGE('',*,*,#3511,.T.);
#4644=ORIENTED_EDGE('',*,*,#3512,.F.);
#4645=ORIENTED_EDGE('',*,*,#3513,.T.);
#4646=ORIENTED_EDGE('',*,*,#3514,.F.);
#4647=ORIENTED_EDGE('',*,*,#3513,.F.);
#4648=ORIENTED_EDGE('',*,*,#3515,.F.);
#4649=ORIENTED_EDGE('',*,*,#3516,.T.);
#4650=ORIENTED_EDGE('',*,*,#3510,.F.);
#4651=ORIENTED_EDGE('',*,*,#3516,.F.);
#4652=ORIENTED_EDGE('',*,*,#3517,.F.);
#4653=ORIENTED_EDGE('',*,*,#3518,.T.);
#4654=ORIENTED_EDGE('',*,*,#3509,.F.);
#4655=ORIENTED_EDGE('',*,*,#3518,.F.);
#4656=ORIENTED_EDGE('',*,*,#3519,.F.);
#4657=ORIENTED_EDGE('',*,*,#3520,.T.);
#4658=ORIENTED_EDGE('',*,*,#3521,.F.);
#4659=ORIENTED_EDGE('',*,*,#3520,.F.);
#4660=ORIENTED_EDGE('',*,*,#3522,.F.);
#4661=ORIENTED_EDGE('',*,*,#3523,.T.);
#4662=ORIENTED_EDGE('',*,*,#3524,.T.);
#4663=ORIENTED_EDGE('',*,*,#3523,.F.);
#4664=ORIENTED_EDGE('',*,*,#3524,.F.);
#4665=ORIENTED_EDGE('',*,*,#3525,.F.);
#4666=ORIENTED_EDGE('',*,*,#3526,.F.);
#4667=ORIENTED_EDGE('',*,*,#3527,.T.);
#4668=ORIENTED_EDGE('',*,*,#3528,.T.);
#4669=ORIENTED_EDGE('',*,*,#3527,.F.);
#4670=ORIENTED_EDGE('',*,*,#3528,.F.);
#4671=ORIENTED_EDGE('',*,*,#3529,.F.);
#4672=ORIENTED_EDGE('',*,*,#3525,.T.);
#4673=ORIENTED_EDGE('',*,*,#3530,.T.);
#4674=ORIENTED_EDGE('',*,*,#3531,.F.);
#4675=ORIENTED_EDGE('',*,*,#3530,.F.);
#4676=ORIENTED_EDGE('',*,*,#3529,.T.);
#4677=ORIENTED_EDGE('',*,*,#3532,.T.);
#4678=ORIENTED_EDGE('',*,*,#3533,.F.);
#4679=ORIENTED_EDGE('',*,*,#3532,.F.);
#4680=ORIENTED_EDGE('',*,*,#3534,.F.);
#4681=ORIENTED_EDGE('',*,*,#3535,.F.);
#4682=ORIENTED_EDGE('',*,*,#3536,.F.);
#4683=ORIENTED_EDGE('',*,*,#3537,.T.);
#4684=ORIENTED_EDGE('',*,*,#3538,.F.);
#4685=ORIENTED_EDGE('',*,*,#3539,.T.);
#4686=ORIENTED_EDGE('',*,*,#3540,.F.);
#4687=ORIENTED_EDGE('',*,*,#3541,.F.);
#4688=ORIENTED_EDGE('',*,*,#3542,.F.);
#4689=ORIENTED_EDGE('',*,*,#3543,.T.);
#4690=ORIENTED_EDGE('',*,*,#3544,.F.);
#4691=ORIENTED_EDGE('',*,*,#3545,.F.);
#4692=ORIENTED_EDGE('',*,*,#3546,.F.);
#4693=ORIENTED_EDGE('',*,*,#3547,.T.);
#4694=ORIENTED_EDGE('',*,*,#3548,.F.);
#4695=ORIENTED_EDGE('',*,*,#3549,.F.);
#4696=ORIENTED_EDGE('',*,*,#3550,.F.);
#4697=ORIENTED_EDGE('',*,*,#3551,.T.);
#4698=ORIENTED_EDGE('',*,*,#3552,.F.);
#4699=ORIENTED_EDGE('',*,*,#3553,.F.);
#4700=ORIENTED_EDGE('',*,*,#3554,.F.);
#4701=ORIENTED_EDGE('',*,*,#3555,.F.);
#4702=ORIENTED_EDGE('',*,*,#3556,.F.);
#4703=ORIENTED_EDGE('',*,*,#3557,.T.);
#4704=ORIENTED_EDGE('',*,*,#3558,.F.);
#4705=ORIENTED_EDGE('',*,*,#3559,.F.);
#4706=ORIENTED_EDGE('',*,*,#3560,.F.);
#4707=ORIENTED_EDGE('',*,*,#3561,.T.);
#4708=ORIENTED_EDGE('',*,*,#3562,.F.);
#4709=ORIENTED_EDGE('',*,*,#3531,.T.);
#4710=ORIENTED_EDGE('',*,*,#3563,.F.);
#4711=ORIENTED_EDGE('',*,*,#3533,.T.);
#4712=ORIENTED_EDGE('',*,*,#3564,.F.);
#4713=ORIENTED_EDGE('',*,*,#3537,.F.);
#4714=ORIENTED_EDGE('',*,*,#3565,.F.);
#4715=ORIENTED_EDGE('',*,*,#3551,.F.);
#4716=ORIENTED_EDGE('',*,*,#3566,.F.);
#4717=ORIENTED_EDGE('',*,*,#3557,.F.);
#4718=ORIENTED_EDGE('',*,*,#3567,.F.);
#4719=ORIENTED_EDGE('',*,*,#3539,.F.);
#4720=ORIENTED_EDGE('',*,*,#3568,.F.);
#4721=ORIENTED_EDGE('',*,*,#3561,.F.);
#4722=ORIENTED_EDGE('',*,*,#3569,.F.);
#4723=ORIENTED_EDGE('',*,*,#3543,.F.);
#4724=ORIENTED_EDGE('',*,*,#3570,.F.);
#4725=ORIENTED_EDGE('',*,*,#3571,.F.);
#4726=ORIENTED_EDGE('',*,*,#3572,.F.);
#4727=ORIENTED_EDGE('',*,*,#3547,.F.);
#4728=ORIENTED_EDGE('',*,*,#3573,.F.);
#4729=ORIENTED_EDGE('',*,*,#3574,.F.);
#4730=ORIENTED_EDGE('',*,*,#3575,.F.);
#4731=ORIENTED_EDGE('',*,*,#3571,.T.);
#4732=ORIENTED_EDGE('',*,*,#3576,.T.);
#4733=ORIENTED_EDGE('',*,*,#3577,.F.);
#4734=ORIENTED_EDGE('',*,*,#3578,.F.);
#4735=ORIENTED_EDGE('',*,*,#3579,.F.);
#4736=ORIENTED_EDGE('',*,*,#3580,.F.);
#4737=ORIENTED_EDGE('',*,*,#3581,.F.);
#4738=ORIENTED_EDGE('',*,*,#3548,.T.);
#4739=ORIENTED_EDGE('',*,*,#3572,.T.);
#4740=ORIENTED_EDGE('',*,*,#3575,.T.);
#4741=ORIENTED_EDGE('',*,*,#3582,.T.);
#4742=ORIENTED_EDGE('',*,*,#3583,.F.);
#4743=ORIENTED_EDGE('',*,*,#3584,.F.);
#4744=ORIENTED_EDGE('',*,*,#3585,.F.);
#4745=ORIENTED_EDGE('',*,*,#3586,.F.);
#4746=ORIENTED_EDGE('',*,*,#3587,.F.);
#4747=ORIENTED_EDGE('',*,*,#3588,.T.);
#4748=ORIENTED_EDGE('',*,*,#3544,.T.);
#4749=ORIENTED_EDGE('',*,*,#3569,.T.);
#4750=ORIENTED_EDGE('',*,*,#3560,.T.);
#4751=ORIENTED_EDGE('',*,*,#3589,.T.);
#4752=ORIENTED_EDGE('',*,*,#3590,.F.);
#4753=ORIENTED_EDGE('',*,*,#3591,.F.);
#4754=ORIENTED_EDGE('',*,*,#3592,.F.);
#4755=ORIENTED_EDGE('',*,*,#3593,.F.);
#4756=ORIENTED_EDGE('',*,*,#3594,.F.);
#4757=ORIENTED_EDGE('',*,*,#3595,.T.);
#4758=ORIENTED_EDGE('',*,*,#3540,.T.);
#4759=ORIENTED_EDGE('',*,*,#3567,.T.);
#4760=ORIENTED_EDGE('',*,*,#3556,.T.);
#4761=ORIENTED_EDGE('',*,*,#3596,.T.);
#4762=ORIENTED_EDGE('',*,*,#3597,.F.);
#4763=ORIENTED_EDGE('',*,*,#3598,.F.);
#4764=ORIENTED_EDGE('',*,*,#3506,.F.);
#4765=ORIENTED_EDGE('',*,*,#3599,.F.);
#4766=ORIENTED_EDGE('',*,*,#3600,.F.);
#4767=ORIENTED_EDGE('',*,*,#3601,.T.);
#4768=ORIENTED_EDGE('',*,*,#3534,.T.);
#4769=ORIENTED_EDGE('',*,*,#3564,.T.);
#4770=ORIENTED_EDGE('',*,*,#3550,.T.);
#4771=ORIENTED_EDGE('',*,*,#3602,.F.);
#4772=ORIENTED_EDGE('',*,*,#3603,.T.);
#4773=ORIENTED_EDGE('',*,*,#3604,.T.);
#4774=ORIENTED_EDGE('',*,*,#3605,.T.);
#4775=ORIENTED_EDGE('',*,*,#3606,.F.);
#4776=ORIENTED_EDGE('',*,*,#3549,.T.);
#4777=ORIENTED_EDGE('',*,*,#3588,.F.);
#4778=ORIENTED_EDGE('',*,*,#3607,.T.);
#4779=ORIENTED_EDGE('',*,*,#3576,.F.);
#4780=ORIENTED_EDGE('',*,*,#3608,.T.);
#4781=ORIENTED_EDGE('',*,*,#3582,.F.);
#4782=ORIENTED_EDGE('',*,*,#3574,.T.);
#4783=ORIENTED_EDGE('',*,*,#3609,.F.);
#4784=ORIENTED_EDGE('',*,*,#3610,.T.);
#4785=ORIENTED_EDGE('',*,*,#3589,.F.);
#4786=ORIENTED_EDGE('',*,*,#3559,.T.);
#4787=ORIENTED_EDGE('',*,*,#3611,.F.);
#4788=ORIENTED_EDGE('',*,*,#3612,.T.);
#4789=ORIENTED_EDGE('',*,*,#3596,.F.);
#4790=ORIENTED_EDGE('',*,*,#3555,.T.);
#4791=ORIENTED_EDGE('',*,*,#3613,.F.);
#4792=ORIENTED_EDGE('',*,*,#3614,.T.);
#4793=ORIENTED_EDGE('',*,*,#3615,.T.);
#4794=ORIENTED_EDGE('',*,*,#3602,.T.);
#4795=ORIENTED_EDGE('',*,*,#3553,.T.);
#4796=ORIENTED_EDGE('',*,*,#3616,.T.);
#4797=ORIENTED_EDGE('',*,*,#3617,.F.);
#4798=ORIENTED_EDGE('',*,*,#3618,.T.);
#4799=ORIENTED_EDGE('',*,*,#3619,.F.);
#4800=ORIENTED_EDGE('',*,*,#3620,.T.);
#4801=ORIENTED_EDGE('',*,*,#3621,.F.);
#4802=ORIENTED_EDGE('',*,*,#3622,.T.);
#4803=ORIENTED_EDGE('',*,*,#3623,.F.);
#4804=ORIENTED_EDGE('',*,*,#3624,.T.);
#4805=ORIENTED_EDGE('',*,*,#3535,.T.);
#4806=ORIENTED_EDGE('',*,*,#3606,.T.);
#4807=ORIENTED_EDGE('',*,*,#3625,.T.);
#4808=ORIENTED_EDGE('',*,*,#3626,.T.);
#4809=ORIENTED_EDGE('',*,*,#3627,.F.);
#4810=ORIENTED_EDGE('',*,*,#3541,.T.);
#4811=ORIENTED_EDGE('',*,*,#3601,.F.);
#4812=ORIENTED_EDGE('',*,*,#3628,.T.);
#4813=ORIENTED_EDGE('',*,*,#3629,.F.);
#4814=ORIENTED_EDGE('',*,*,#3545,.T.);
#4815=ORIENTED_EDGE('',*,*,#3595,.F.);
#4816=ORIENTED_EDGE('',*,*,#3630,.T.);
#4817=ORIENTED_EDGE('',*,*,#3631,.F.);
#4818=ORIENTED_EDGE('',*,*,#3632,.T.);
#4819=ORIENTED_EDGE('',*,*,#3633,.T.);
#4820=ORIENTED_EDGE('',*,*,#3634,.T.);
#4821=ORIENTED_EDGE('',*,*,#3635,.T.);
#4822=ORIENTED_EDGE('',*,*,#3636,.T.);
#4823=ORIENTED_EDGE('',*,*,#3637,.F.);
#4824=ORIENTED_EDGE('',*,*,#3638,.F.);
#4825=ORIENTED_EDGE('',*,*,#3639,.T.);
#4826=ORIENTED_EDGE('',*,*,#3563,.T.);
#4827=ORIENTED_EDGE('',*,*,#3639,.F.);
#4828=ORIENTED_EDGE('',*,*,#3511,.F.);
#4829=ORIENTED_EDGE('',*,*,#3640,.T.);
#4830=ORIENTED_EDGE('',*,*,#3562,.T.);
#4831=ORIENTED_EDGE('',*,*,#3640,.F.);
#4832=ORIENTED_EDGE('',*,*,#3641,.F.);
#4833=ORIENTED_EDGE('',*,*,#3637,.T.);
#4834=ORIENTED_EDGE('',*,*,#3642,.F.);
#4835=ORIENTED_EDGE('',*,*,#3643,.F.);
#4836=ORIENTED_EDGE('',*,*,#3644,.F.);
#4837=ORIENTED_EDGE('',*,*,#3645,.F.);
#4838=ORIENTED_EDGE('',*,*,#3577,.T.);
#4839=ORIENTED_EDGE('',*,*,#3607,.F.);
#4840=ORIENTED_EDGE('',*,*,#3587,.T.);
#4841=ORIENTED_EDGE('',*,*,#3646,.T.);
#4842=ORIENTED_EDGE('',*,*,#3641,.T.);
#4843=ORIENTED_EDGE('',*,*,#3647,.T.);
#4844=ORIENTED_EDGE('',*,*,#3648,.T.);
#4845=ORIENTED_EDGE('',*,*,#3632,.F.);
#4846=ORIENTED_EDGE('',*,*,#3578,.T.);
#4847=ORIENTED_EDGE('',*,*,#3646,.F.);
#4848=ORIENTED_EDGE('',*,*,#3586,.T.);
#4849=ORIENTED_EDGE('',*,*,#3649,.F.);
#4850=ORIENTED_EDGE('',*,*,#3645,.T.);
#4851=ORIENTED_EDGE('',*,*,#3650,.F.);
#4852=ORIENTED_EDGE('',*,*,#3651,.F.);
#4853=ORIENTED_EDGE('',*,*,#3647,.F.);
#4854=ORIENTED_EDGE('',*,*,#3579,.T.);
#4855=ORIENTED_EDGE('',*,*,#3649,.T.);
#4856=ORIENTED_EDGE('',*,*,#3585,.T.);
#4857=ORIENTED_EDGE('',*,*,#3652,.T.);
#4858=ORIENTED_EDGE('',*,*,#3514,.T.);
#4859=ORIENTED_EDGE('',*,*,#3521,.T.);
#4860=ORIENTED_EDGE('',*,*,#3638,.T.);
#4861=ORIENTED_EDGE('',*,*,#3644,.T.);
#4862=ORIENTED_EDGE('',*,*,#3653,.T.);
#4863=ORIENTED_EDGE('',*,*,#3654,.T.);
#4864=ORIENTED_EDGE('',*,*,#3650,.T.);
#4865=ORIENTED_EDGE('',*,*,#3580,.T.);
#4866=ORIENTED_EDGE('',*,*,#3652,.F.);
#4867=ORIENTED_EDGE('',*,*,#3584,.T.);
#4868=ORIENTED_EDGE('',*,*,#3655,.F.);
#4869=ORIENTED_EDGE('',*,*,#3581,.T.);
#4870=ORIENTED_EDGE('',*,*,#3655,.T.);
#4871=ORIENTED_EDGE('',*,*,#3583,.T.);
#4872=ORIENTED_EDGE('',*,*,#3608,.F.);
#4873=ORIENTED_EDGE('',*,*,#3642,.T.);
#4874=ORIENTED_EDGE('',*,*,#3636,.F.);
#4875=ORIENTED_EDGE('',*,*,#3656,.T.);
#4876=ORIENTED_EDGE('',*,*,#3657,.T.);
#4877=ORIENTED_EDGE('',*,*,#3546,.T.);
#4878=ORIENTED_EDGE('',*,*,#3631,.T.);
#4879=ORIENTED_EDGE('',*,*,#3658,.F.);
#4880=ORIENTED_EDGE('',*,*,#3659,.F.);
#4881=ORIENTED_EDGE('',*,*,#3660,.F.);
#4882=ORIENTED_EDGE('',*,*,#3661,.F.);
#4883=ORIENTED_EDGE('',*,*,#3662,.F.);
#4884=ORIENTED_EDGE('',*,*,#3609,.T.);
#4885=ORIENTED_EDGE('',*,*,#3573,.T.);
#4886=ORIENTED_EDGE('',*,*,#3570,.T.);
#4887=ORIENTED_EDGE('',*,*,#3658,.T.);
#4888=ORIENTED_EDGE('',*,*,#3630,.F.);
#4889=ORIENTED_EDGE('',*,*,#3594,.T.);
#4890=ORIENTED_EDGE('',*,*,#3663,.T.);
#4891=ORIENTED_EDGE('',*,*,#3659,.T.);
#4892=ORIENTED_EDGE('',*,*,#3663,.F.);
#4893=ORIENTED_EDGE('',*,*,#3593,.T.);
#4894=ORIENTED_EDGE('',*,*,#3664,.F.);
#4895=ORIENTED_EDGE('',*,*,#3660,.T.);
#4896=ORIENTED_EDGE('',*,*,#3664,.T.);
#4897=ORIENTED_EDGE('',*,*,#3592,.T.);
#4898=ORIENTED_EDGE('',*,*,#3665,.T.);
#4899=ORIENTED_EDGE('',*,*,#3661,.T.);
#4900=ORIENTED_EDGE('',*,*,#3665,.F.);
#4901=ORIENTED_EDGE('',*,*,#3591,.T.);
#4902=ORIENTED_EDGE('',*,*,#3666,.F.);
#4903=ORIENTED_EDGE('',*,*,#3662,.T.);
#4904=ORIENTED_EDGE('',*,*,#3666,.T.);
#4905=ORIENTED_EDGE('',*,*,#3590,.T.);
#4906=ORIENTED_EDGE('',*,*,#3610,.F.);
#4907=ORIENTED_EDGE('',*,*,#3542,.T.);
#4908=ORIENTED_EDGE('',*,*,#3629,.T.);
#4909=ORIENTED_EDGE('',*,*,#3667,.F.);
#4910=ORIENTED_EDGE('',*,*,#3668,.F.);
#4911=ORIENTED_EDGE('',*,*,#3502,.F.);
#4912=ORIENTED_EDGE('',*,*,#3669,.F.);
#4913=ORIENTED_EDGE('',*,*,#3670,.F.);
#4914=ORIENTED_EDGE('',*,*,#3611,.T.);
#4915=ORIENTED_EDGE('',*,*,#3558,.T.);
#4916=ORIENTED_EDGE('',*,*,#3568,.T.);
#4917=ORIENTED_EDGE('',*,*,#3667,.T.);
#4918=ORIENTED_EDGE('',*,*,#3628,.F.);
#4919=ORIENTED_EDGE('',*,*,#3600,.T.);
#4920=ORIENTED_EDGE('',*,*,#3671,.T.);
#4921=ORIENTED_EDGE('',*,*,#3504,.T.);
#4922=ORIENTED_EDGE('',*,*,#3503,.F.);
#4923=ORIENTED_EDGE('',*,*,#3668,.T.);
#4924=ORIENTED_EDGE('',*,*,#3671,.F.);
#4925=ORIENTED_EDGE('',*,*,#3599,.T.);
#4926=ORIENTED_EDGE('',*,*,#3505,.F.);
#4927=ORIENTED_EDGE('',*,*,#3508,.T.);
#4928=ORIENTED_EDGE('',*,*,#3507,.F.);
#4929=ORIENTED_EDGE('',*,*,#3598,.T.);
#4930=ORIENTED_EDGE('',*,*,#3672,.F.);
#4931=ORIENTED_EDGE('',*,*,#3669,.T.);
#4932=ORIENTED_EDGE('',*,*,#3501,.F.);
#4933=ORIENTED_EDGE('',*,*,#3670,.T.);
#4934=ORIENTED_EDGE('',*,*,#3672,.T.);
#4935=ORIENTED_EDGE('',*,*,#3597,.T.);
#4936=ORIENTED_EDGE('',*,*,#3612,.F.);
#4937=ORIENTED_EDGE('',*,*,#3538,.T.);
#4938=ORIENTED_EDGE('',*,*,#3627,.T.);
#4939=ORIENTED_EDGE('',*,*,#3673,.F.);
#4940=ORIENTED_EDGE('',*,*,#3674,.F.);
#4941=ORIENTED_EDGE('',*,*,#3675,.F.);
#4942=ORIENTED_EDGE('',*,*,#3676,.F.);
#4943=ORIENTED_EDGE('',*,*,#3677,.F.);
#4944=ORIENTED_EDGE('',*,*,#3613,.T.);
#4945=ORIENTED_EDGE('',*,*,#3554,.T.);
#4946=ORIENTED_EDGE('',*,*,#3566,.T.);
#4947=ORIENTED_EDGE('',*,*,#3673,.T.);
#4948=ORIENTED_EDGE('',*,*,#3626,.F.);
#4949=ORIENTED_EDGE('',*,*,#3678,.T.);
#4950=ORIENTED_EDGE('',*,*,#3679,.T.);
#4951=ORIENTED_EDGE('',*,*,#3674,.T.);
#4952=ORIENTED_EDGE('',*,*,#3679,.F.);
#4953=ORIENTED_EDGE('',*,*,#3680,.F.);
#4954=ORIENTED_EDGE('',*,*,#3681,.F.);
#4955=ORIENTED_EDGE('',*,*,#3675,.T.);
#4956=ORIENTED_EDGE('',*,*,#3681,.T.);
#4957=ORIENTED_EDGE('',*,*,#3682,.T.);
#4958=ORIENTED_EDGE('',*,*,#3683,.T.);
#4959=ORIENTED_EDGE('',*,*,#3677,.T.);
#4960=ORIENTED_EDGE('',*,*,#3684,.T.);
#4961=ORIENTED_EDGE('',*,*,#3685,.T.);
#4962=ORIENTED_EDGE('',*,*,#3614,.F.);
#4963=ORIENTED_EDGE('',*,*,#3676,.T.);
#4964=ORIENTED_EDGE('',*,*,#3683,.F.);
#4965=ORIENTED_EDGE('',*,*,#3686,.F.);
#4966=ORIENTED_EDGE('',*,*,#3684,.F.);
#4967=ORIENTED_EDGE('',*,*,#3687,.T.);
#4968=ORIENTED_EDGE('',*,*,#3688,.T.);
#4969=ORIENTED_EDGE('',*,*,#3686,.T.);
#4970=ORIENTED_EDGE('',*,*,#3689,.T.);
#4971=ORIENTED_EDGE('',*,*,#3690,.T.);
#4972=ORIENTED_EDGE('',*,*,#3691,.T.);
#4973=ORIENTED_EDGE('',*,*,#3680,.T.);
#4974=ORIENTED_EDGE('',*,*,#3692,.T.);
#4975=ORIENTED_EDGE('',*,*,#3693,.T.);
#4976=ORIENTED_EDGE('',*,*,#3687,.F.);
#4977=ORIENTED_EDGE('',*,*,#3682,.F.);
#4978=ORIENTED_EDGE('',*,*,#3693,.F.);
#4979=ORIENTED_EDGE('',*,*,#3604,.F.);
#4980=ORIENTED_EDGE('',*,*,#3625,.F.);
#4981=ORIENTED_EDGE('',*,*,#3605,.F.);
#4982=ORIENTED_EDGE('',*,*,#3692,.F.);
#4983=ORIENTED_EDGE('',*,*,#3678,.F.);
#4984=ORIENTED_EDGE('',*,*,#3694,.T.);
#4985=ORIENTED_EDGE('',*,*,#3651,.T.);
#4986=ORIENTED_EDGE('',*,*,#3695,.T.);
#4987=ORIENTED_EDGE('',*,*,#3695,.F.);
#4988=ORIENTED_EDGE('',*,*,#3654,.F.);
#4989=ORIENTED_EDGE('',*,*,#3691,.F.);
#4990=ORIENTED_EDGE('',*,*,#3696,.F.);
#4991=ORIENTED_EDGE('',*,*,#3633,.F.);
#4992=ORIENTED_EDGE('',*,*,#3648,.F.);
#4993=ORIENTED_EDGE('',*,*,#3694,.F.);
#4994=ORIENTED_EDGE('',*,*,#3697,.F.);
#4995=ORIENTED_EDGE('',*,*,#3635,.F.);
#4996=ORIENTED_EDGE('',*,*,#3698,.F.);
#4997=ORIENTED_EDGE('',*,*,#3690,.F.);
#4998=ORIENTED_EDGE('',*,*,#3656,.F.);
#4999=ORIENTED_EDGE('',*,*,#3643,.T.);
#5000=ORIENTED_EDGE('',*,*,#3657,.F.);
#5001=ORIENTED_EDGE('',*,*,#3689,.F.);
#5002=ORIENTED_EDGE('',*,*,#3653,.F.);
#5003=ORIENTED_EDGE('',*,*,#3615,.F.);
#5004=ORIENTED_EDGE('',*,*,#3685,.F.);
#5005=ORIENTED_EDGE('',*,*,#3688,.F.);
#5006=ORIENTED_EDGE('',*,*,#3603,.F.);
#5007=ORIENTED_EDGE('',*,*,#3697,.T.);
#5008=ORIENTED_EDGE('',*,*,#3696,.T.);
#5009=ORIENTED_EDGE('',*,*,#3698,.T.);
#5010=ORIENTED_EDGE('',*,*,#3634,.F.);
#5011=ORIENTED_EDGE('',*,*,#3699,.F.);
#5012=ORIENTED_EDGE('',*,*,#3700,.F.);
#5013=ORIENTED_EDGE('',*,*,#3701,.F.);
#5014=ORIENTED_EDGE('',*,*,#3702,.F.);
#5015=ORIENTED_EDGE('',*,*,#3703,.F.);
#5016=ORIENTED_EDGE('',*,*,#3704,.F.);
#5017=ORIENTED_EDGE('',*,*,#3705,.F.);
#5018=ORIENTED_EDGE('',*,*,#3706,.F.);
#5019=ORIENTED_EDGE('',*,*,#3707,.F.);
#5020=ORIENTED_EDGE('',*,*,#3699,.T.);
#5021=ORIENTED_EDGE('',*,*,#3708,.T.);
#5022=ORIENTED_EDGE('',*,*,#3706,.T.);
#5023=ORIENTED_EDGE('',*,*,#3709,.T.);
#5024=ORIENTED_EDGE('',*,*,#3623,.T.);
#5025=ORIENTED_EDGE('',*,*,#3710,.T.);
#5026=ORIENTED_EDGE('',*,*,#3707,.T.);
#5027=ORIENTED_EDGE('',*,*,#3711,.T.);
#5028=ORIENTED_EDGE('',*,*,#3712,.F.);
#5029=ORIENTED_EDGE('',*,*,#3713,.F.);
#5030=ORIENTED_EDGE('',*,*,#3714,.F.);
#5031=ORIENTED_EDGE('',*,*,#3713,.T.);
#5032=ORIENTED_EDGE('',*,*,#3715,.T.);
#5033=ORIENTED_EDGE('',*,*,#3703,.T.);
#5034=ORIENTED_EDGE('',*,*,#3716,.T.);
#5035=ORIENTED_EDGE('',*,*,#3705,.T.);
#5036=ORIENTED_EDGE('',*,*,#3717,.T.);
#5037=ORIENTED_EDGE('',*,*,#3714,.T.);
#5038=ORIENTED_EDGE('',*,*,#3718,.T.);
#5039=ORIENTED_EDGE('',*,*,#3621,.T.);
#5040=ORIENTED_EDGE('',*,*,#3719,.T.);
#5041=ORIENTED_EDGE('',*,*,#3712,.T.);
#5042=ORIENTED_EDGE('',*,*,#3720,.T.);
#5043=ORIENTED_EDGE('',*,*,#3619,.T.);
#5044=ORIENTED_EDGE('',*,*,#3721,.T.);
#5045=ORIENTED_EDGE('',*,*,#3704,.T.);
#5046=ORIENTED_EDGE('',*,*,#3722,.T.);
#5047=ORIENTED_EDGE('',*,*,#3702,.T.);
#5048=ORIENTED_EDGE('',*,*,#3723,.T.);
#5049=ORIENTED_EDGE('',*,*,#3700,.T.);
#5050=ORIENTED_EDGE('',*,*,#3724,.T.);
#5051=ORIENTED_EDGE('',*,*,#3617,.T.);
#5052=ORIENTED_EDGE('',*,*,#3725,.T.);
#5053=ORIENTED_EDGE('',*,*,#3701,.T.);
#5054=ORIENTED_EDGE('',*,*,#3726,.T.);
#5055=ORIENTED_EDGE('',*,*,#3720,.F.);
#5056=ORIENTED_EDGE('',*,*,#3717,.F.);
#5057=ORIENTED_EDGE('',*,*,#3710,.F.);
#5058=ORIENTED_EDGE('',*,*,#3622,.F.);
#5059=ORIENTED_EDGE('',*,*,#3536,.T.);
#5060=ORIENTED_EDGE('',*,*,#3624,.F.);
#5061=ORIENTED_EDGE('',*,*,#3711,.F.);
#5062=ORIENTED_EDGE('',*,*,#3708,.F.);
#5063=ORIENTED_EDGE('',*,*,#3725,.F.);
#5064=ORIENTED_EDGE('',*,*,#3616,.F.);
#5065=ORIENTED_EDGE('',*,*,#3552,.T.);
#5066=ORIENTED_EDGE('',*,*,#3565,.T.);
#5067=ORIENTED_EDGE('',*,*,#3716,.F.);
#5068=ORIENTED_EDGE('',*,*,#3724,.F.);
#5069=ORIENTED_EDGE('',*,*,#3709,.F.);
#5070=ORIENTED_EDGE('',*,*,#3718,.F.);
#5071=ORIENTED_EDGE('',*,*,#3526,.T.);
#5072=ORIENTED_EDGE('',*,*,#3522,.T.);
#5073=ORIENTED_EDGE('',*,*,#3519,.T.);
#5074=ORIENTED_EDGE('',*,*,#3517,.T.);
#5075=ORIENTED_EDGE('',*,*,#3515,.T.);
#5076=ORIENTED_EDGE('',*,*,#3512,.T.);
#5077=ORIENTED_EDGE('',*,*,#3721,.F.);
#5078=ORIENTED_EDGE('',*,*,#3618,.F.);
#5079=ORIENTED_EDGE('',*,*,#3726,.F.);
#5080=ORIENTED_EDGE('',*,*,#3723,.F.);
#5081=ORIENTED_EDGE('',*,*,#3719,.F.);
#5082=ORIENTED_EDGE('',*,*,#3620,.F.);
#5083=ORIENTED_EDGE('',*,*,#3722,.F.);
#5084=ORIENTED_EDGE('',*,*,#3715,.F.);
#6317=CYLINDRICAL_SURFACE('',#7046,0.15);
#6318=CYLINDRICAL_SURFACE('',#7049,0.15);
#6319=CYLINDRICAL_SURFACE('',#7051,0.15);
#6320=CYLINDRICAL_SURFACE('',#7053,0.15);
#6321=CYLINDRICAL_SURFACE('',#7056,0.3);
#6322=CYLINDRICAL_SURFACE('',#7061,0.3);
#6323=CYLINDRICAL_SURFACE('',#7066,0.17);
#6324=CYLINDRICAL_SURFACE('',#7068,0.17);
#6325=CYLINDRICAL_SURFACE('',#7092,0.4);
#6326=CYLINDRICAL_SURFACE('',#7094,0.4);
#6327=CYLINDRICAL_SURFACE('',#7116,0.1);
#6328=CYLINDRICAL_SURFACE('',#7120,0.1);
#6329=CYLINDRICAL_SURFACE('',#7134,0.3);
#6330=CYLINDRICAL_SURFACE('',#7139,0.3);
#6494=ADVANCED_FACE('',(#875,#601,#602,#603),#699,.F.);
#6495=ADVANCED_FACE('',(#876),#6317,.F.);
#6496=ADVANCED_FACE('',(#877),#6318,.F.);
#6497=ADVANCED_FACE('',(#878),#6319,.F.);
#6498=ADVANCED_FACE('',(#879),#6320,.F.);
#6499=ADVANCED_FACE('',(#880),#6321,.F.);
#6500=ADVANCED_FACE('',(#881,#604),#700,.F.);
#6501=ADVANCED_FACE('',(#882),#6322,.F.);
#6502=ADVANCED_FACE('',(#883,#605),#701,.F.);
#6503=ADVANCED_FACE('',(#884),#6323,.F.);
#6504=ADVANCED_FACE('',(#885),#6324,.F.);
#6505=ADVANCED_FACE('',(#886),#702,.F.);
#6506=ADVANCED_FACE('',(#887),#703,.F.);
#6507=ADVANCED_FACE('',(#888),#704,.F.);
#6508=ADVANCED_FACE('',(#889),#705,.F.);
#6509=ADVANCED_FACE('',(#890),#706,.F.);
#6510=ADVANCED_FACE('',(#891),#707,.F.);
#6511=ADVANCED_FACE('',(#892),#708,.F.);
#6512=ADVANCED_FACE('',(#893,#606),#709,.F.);
#6513=ADVANCED_FACE('',(#894,#607),#710,.F.);
#6514=ADVANCED_FACE('',(#895),#711,.F.);
#6515=ADVANCED_FACE('',(#896),#712,.F.);
#6516=ADVANCED_FACE('',(#897),#713,.F.);
#6517=ADVANCED_FACE('',(#898),#714,.F.);
#6518=ADVANCED_FACE('',(#899),#715,.F.);
#6519=ADVANCED_FACE('',(#900),#716,.T.);
#6520=ADVANCED_FACE('',(#901),#717,.T.);
#6521=ADVANCED_FACE('',(#902),#718,.T.);
#6522=ADVANCED_FACE('',(#903),#719,.T.);
#6523=ADVANCED_FACE('',(#904),#720,.T.);
#6524=ADVANCED_FACE('',(#905,#608),#721,.F.);
#6525=ADVANCED_FACE('',(#906),#6325,.T.);
#6526=ADVANCED_FACE('',(#907),#6326,.T.);
#6527=ADVANCED_FACE('',(#908),#722,.T.);
#6528=ADVANCED_FACE('',(#909),#92,.T.);
#6529=ADVANCED_FACE('',(#910),#93,.T.);
#6530=ADVANCED_FACE('',(#911),#94,.T.);
#6531=ADVANCED_FACE('',(#912),#95,.T.);
#6532=ADVANCED_FACE('',(#913,#609,#610,#611),#723,.F.);
#6533=ADVANCED_FACE('',(#914),#724,.F.);
#6534=ADVANCED_FACE('',(#915),#96,.T.);
#6535=ADVANCED_FACE('',(#916),#97,.T.);
#6536=ADVANCED_FACE('',(#917),#98,.T.);
#6537=ADVANCED_FACE('',(#918),#725,.T.);
#6538=ADVANCED_FACE('',(#919),#99,.T.);
#6539=ADVANCED_FACE('',(#920),#100,.T.);
#6540=ADVANCED_FACE('',(#921),#726,.F.);
#6541=ADVANCED_FACE('',(#922),#101,.T.);
#6542=ADVANCED_FACE('',(#923),#102,.T.);
#6543=ADVANCED_FACE('',(#924),#727,.T.);
#6544=ADVANCED_FACE('',(#925),#103,.T.);
#6545=ADVANCED_FACE('',(#926),#104,.T.);
#6546=ADVANCED_FACE('',(#927),#105,.T.);
#6547=ADVANCED_FACE('',(#928),#106,.T.);
#6548=ADVANCED_FACE('',(#929),#728,.T.);
#6549=ADVANCED_FACE('',(#930),#107,.T.);
#6550=ADVANCED_FACE('',(#931),#108,.T.);
#6551=ADVANCED_FACE('',(#932),#729,.F.);
#6552=ADVANCED_FACE('',(#933),#109,.T.);
#6553=ADVANCED_FACE('',(#934),#110,.T.);
#6554=ADVANCED_FACE('',(#935),#76,.F.);
#6555=ADVANCED_FACE('',(#936),#77,.F.);
#6556=ADVANCED_FACE('',(#937),#78,.F.);
#6557=ADVANCED_FACE('',(#938),#6327,.F.);
#6558=ADVANCED_FACE('',(#939),#111,.T.);
#6559=ADVANCED_FACE('',(#940),#79,.F.);
#6560=ADVANCED_FACE('',(#941),#6328,.F.);
#6561=ADVANCED_FACE('',(#942),#112,.T.);
#6562=ADVANCED_FACE('',(#943),#113,.T.);
#6563=ADVANCED_FACE('',(#944),#114,.T.);
#6564=ADVANCED_FACE('',(#945),#115,.T.);
#6565=ADVANCED_FACE('',(#946),#730,.T.);
#6566=ADVANCED_FACE('',(#947),#80,.T.);
#6567=ADVANCED_FACE('',(#948),#81,.T.);
#6568=ADVANCED_FACE('',(#949),#82,.T.);
#6569=ADVANCED_FACE('',(#950),#6329,.T.);
#6570=ADVANCED_FACE('',(#951),#116,.F.);
#6571=ADVANCED_FACE('',(#952),#83,.T.);
#6572=ADVANCED_FACE('',(#953),#6330,.T.);
#6573=ADVANCED_FACE('',(#954),#117,.F.);
#6574=ADVANCED_FACE('',(#955),#118,.F.);
#6575=ADVANCED_FACE('',(#956),#119,.F.);
#6576=ADVANCED_FACE('',(#957),#120,.F.);
#6577=ADVANCED_FACE('',(#958),#121,.F.);
#6578=ADVANCED_FACE('',(#959),#122,.F.);
#6579=ADVANCED_FACE('',(#960),#731,.F.);
#6580=ADVANCED_FACE('',(#961,#612,#613,#614,#615,#616,#617),#732,.T.);
#6581=ADVANCED_FACE('',(#962),#123,.F.);
#6582=ADVANCED_FACE('',(#963),#733,.F.);
#6824=CLOSED_SHELL('',(#6494,#6495,#6496,#6497,#6498,#6499,#6500,#6501,
#6502,#6503,#6504,#6505,#6506,#6507,#6508,#6509,#6510,#6511,#6512,#6513,
#6514,#6515,#6516,#6517,#6518,#6519,#6520,#6521,#6522,#6523,#6524,#6525,
#6526,#6527,#6528,#6529,#6530,#6531,#6532,#6533,#6534,#6535,#6536,#6537,
#6538,#6539,#6540,#6541,#6542,#6543,#6544,#6545,#6546,#6547,#6548,#6549,
#6550,#6551,#6552,#6553,#6554,#6555,#6556,#6557,#6558,#6559,#6560,#6561,
#6562,#6563,#6564,#6565,#6566,#6567,#6568,#6569,#6570,#6571,#6572,#6573,
#6574,#6575,#6576,#6577,#6578,#6579,#6580,#6581,#6582));
#7041=AXIS2_PLACEMENT_3D('',#9193,#7754,#7755);
#7042=AXIS2_PLACEMENT_3D('',#9194,#7756,#7757);
#7043=AXIS2_PLACEMENT_3D('',#9260,#7760,#7761);
#7044=AXIS2_PLACEMENT_3D('',#9262,#7762,#7763);
#7045=AXIS2_PLACEMENT_3D('',#9264,#7764,#7765);
#7046=AXIS2_PLACEMENT_3D('',#9265,#7766,#7767);
#7047=AXIS2_PLACEMENT_3D('',#9267,#7768,#7769);
#7048=AXIS2_PLACEMENT_3D('',#9270,#7771,#7772);
#7049=AXIS2_PLACEMENT_3D('',#9271,#7773,#7774);
#7050=AXIS2_PLACEMENT_3D('',#9273,#7775,#7776);
#7051=AXIS2_PLACEMENT_3D('',#9275,#7778,#7779);
#7052=AXIS2_PLACEMENT_3D('',#9277,#7780,#7781);
#7053=AXIS2_PLACEMENT_3D('',#9279,#7783,#7784);
#7054=AXIS2_PLACEMENT_3D('',#9281,#7785,#7786);
#7055=AXIS2_PLACEMENT_3D('',#9284,#7788,#7789);
#7056=AXIS2_PLACEMENT_3D('',#9285,#7790,#7791);
#7057=AXIS2_PLACEMENT_3D('',#9287,#7792,#7793);
#7058=AXIS2_PLACEMENT_3D('',#9290,#7795,#7796);
#7059=AXIS2_PLACEMENT_3D('',#9291,#7797,#7798);
#7060=AXIS2_PLACEMENT_3D('',#9293,#7799,#7800);
#7061=AXIS2_PLACEMENT_3D('',#9294,#7801,#7802);
#7062=AXIS2_PLACEMENT_3D('',#9296,#7803,#7804);
#7063=AXIS2_PLACEMENT_3D('',#9299,#7806,#7807);
#7064=AXIS2_PLACEMENT_3D('',#9300,#7808,#7809);
#7065=AXIS2_PLACEMENT_3D('',#9302,#7810,#7811);
#7066=AXIS2_PLACEMENT_3D('',#9303,#7812,#7813);
#7067=AXIS2_PLACEMENT_3D('',#9306,#7815,#7816);
#7068=AXIS2_PLACEMENT_3D('',#9307,#7817,#7818);
#7069=AXIS2_PLACEMENT_3D('',#9310,#7820,#7821);
#7070=AXIS2_PLACEMENT_3D('',#9311,#7822,#7823);
#7071=AXIS2_PLACEMENT_3D('',#9320,#7828,#7829);
#7072=AXIS2_PLACEMENT_3D('',#9329,#7834,#7835);
#7073=AXIS2_PLACEMENT_3D('',#9338,#7840,#7841);
#7074=AXIS2_PLACEMENT_3D('',#9347,#7846,#7847);
#7075=AXIS2_PLACEMENT_3D('',#9356,#7852,#7853);
#7076=AXIS2_PLACEMENT_3D('',#9365,#7858,#7859);
#7077=AXIS2_PLACEMENT_3D('',#9374,#7864,#7865);
#7078=AXIS2_PLACEMENT_3D('',#9376,#7866,#7867);
#7079=AXIS2_PLACEMENT_3D('',#9377,#7868,#7869);
#7080=AXIS2_PLACEMENT_3D('',#9379,#7870,#7871);
#7081=AXIS2_PLACEMENT_3D('',#9380,#7872,#7873);
#7082=AXIS2_PLACEMENT_3D('',#9383,#7876,#7877);
#7083=AXIS2_PLACEMENT_3D('',#9386,#7880,#7881);
#7084=AXIS2_PLACEMENT_3D('',#9389,#7884,#7885);
#7085=AXIS2_PLACEMENT_3D('',#9395,#7889,#7890);
#7086=AXIS2_PLACEMENT_3D('',#9401,#7894,#7895);
#7087=AXIS2_PLACEMENT_3D('',#9478,#7898,#7899);
#7088=AXIS2_PLACEMENT_3D('',#9556,#7903,#7904);
#7089=AXIS2_PLACEMENT_3D('',#9634,#7908,#7909);
#7090=AXIS2_PLACEMENT_3D('',#9709,#7912,#7913);
#7091=AXIS2_PLACEMENT_3D('',#9725,#7917,#7918);
#7092=AXIS2_PLACEMENT_3D('',#10103,#7930,#7931);
#7093=AXIS2_PLACEMENT_3D('',#10105,#7932,#7933);
#7094=AXIS2_PLACEMENT_3D('',#10107,#7935,#7936);
#7095=AXIS2_PLACEMENT_3D('',#10109,#7938,#7939);
#7096=AXIS2_PLACEMENT_3D('',#10277,#7941,#7942);
#7097=AXIS2_PLACEMENT_3D('',#10278,#7943,#7944);
#7098=AXIS2_PLACEMENT_3D('',#10283,#7945,#7946);
#7099=AXIS2_PLACEMENT_3D('',#10355,#7948,#7949);
#7100=AXIS2_PLACEMENT_3D('',#10473,#7951,#7952);
#7101=AXIS2_PLACEMENT_3D('',#10518,#7953,#7954);
#7102=AXIS2_PLACEMENT_3D('',#10669,#7955,#7956);
#7103=AXIS2_PLACEMENT_3D('',#10789,#7958,#7959);
#7104=AXIS2_PLACEMENT_3D('',#10794,#7960,#7961);
#7105=AXIS2_PLACEMENT_3D('',#10846,#7963,#7964);
#7106=AXIS2_PLACEMENT_3D('',#10847,#7965,#7966);
#7107=AXIS2_PLACEMENT_3D('',#10848,#7967,#7968);
#7108=AXIS2_PLACEMENT_3D('',#10849,#7969,#7970);
#7109=AXIS2_PLACEMENT_3D('',#10850,#7971,#7972);
#7110=AXIS2_PLACEMENT_3D('',#10851,#7973,#7974);
#7111=AXIS2_PLACEMENT_3D('',#10853,#7975,#7976);
#7112=AXIS2_PLACEMENT_3D('',#10854,#7977,#7978);
#7113=AXIS2_PLACEMENT_3D('',#10855,#7979,#7980);
#7114=AXIS2_PLACEMENT_3D('',#10856,#7981,#7982);
#7115=AXIS2_PLACEMENT_3D('',#10857,#7983,#7984);
#7116=AXIS2_PLACEMENT_3D('',#10858,#7985,#7986);
#7117=AXIS2_PLACEMENT_3D('',#10879,#7987,#7988);
#7118=AXIS2_PLACEMENT_3D('',#10881,#7989,#7990);
#7119=AXIS2_PLACEMENT_3D('',#10882,#7991,#7992);
#7120=AXIS2_PLACEMENT_3D('',#10883,#7993,#7994);
#7121=AXIS2_PLACEMENT_3D('',#10981,#7996,#7997);
#7122=AXIS2_PLACEMENT_3D('',#10982,#7998,#7999);
#7123=AXIS2_PLACEMENT_3D('',#10985,#8000,#8001);
#7124=AXIS2_PLACEMENT_3D('',#10987,#8002,#8003);
#7125=AXIS2_PLACEMENT_3D('',#10988,#8004,#8005);
#7126=AXIS2_PLACEMENT_3D('',#10989,#8006,#8007);
#7127=AXIS2_PLACEMENT_3D('',#10992,#8008,#8009);
#7128=AXIS2_PLACEMENT_3D('',#10994,#8010,#8011);
#7129=AXIS2_PLACEMENT_3D('',#10995,#8012,#8013);
#7130=AXIS2_PLACEMENT_3D('',#10996,#8014,#8015);
#7131=AXIS2_PLACEMENT_3D('',#10999,#8016,#8017);
#7132=AXIS2_PLACEMENT_3D('',#11001,#8018,#8019);
#7133=AXIS2_PLACEMENT_3D('',#11002,#8020,#8021);
#7134=AXIS2_PLACEMENT_3D('',#11003,#8022,#8023);
#7135=AXIS2_PLACEMENT_3D('',#11034,#8026,#8027);
#7136=AXIS2_PLACEMENT_3D('',#11037,#8028,#8029);
#7137=AXIS2_PLACEMENT_3D('',#11039,#8030,#8031);
#7138=AXIS2_PLACEMENT_3D('',#11040,#8032,#8033);
#7139=AXIS2_PLACEMENT_3D('',#11041,#8034,#8035);
#7140=AXIS2_PLACEMENT_3D('',#11222,#8038,#8039);
#7141=AXIS2_PLACEMENT_3D('',#11223,#8040,#8041);
#7142=AXIS2_PLACEMENT_3D('',#11240,#8042,#8043);
#7754=DIRECTION('axis',(0.,0.,1.));
#7755=DIRECTION('refdir',(1.,0.,0.));
#7756=DIRECTION('center_axis',(-9.61618982193066E-33,1.03600583455278E-18,
1.));
#7757=DIRECTION('ref_axis',(1.,0.,9.61618982193066E-33));
#7758=DIRECTION('',(0.,-1.,1.03600583455278E-18));
#7759=DIRECTION('',(0.,1.,-1.03600583455278E-18));
#7760=DIRECTION('center_axis',(-9.61618982193066E-33,1.03600583455278E-18,
1.));
#7761=DIRECTION('ref_axis',(1.,0.,0.));
#7762=DIRECTION('center_axis',(-9.61618982193066E-33,1.03600583455278E-18,
1.));
#7763=DIRECTION('ref_axis',(1.,0.,0.));
#7764=DIRECTION('center_axis',(-9.61618982193066E-33,1.03600583455278E-18,
1.));
#7765=DIRECTION('ref_axis',(1.,0.,0.));
#7766=DIRECTION('center_axis',(0.,0.,-1.));
#7767=DIRECTION('ref_axis',(1.,0.,0.));
#7768=DIRECTION('center_axis',(9.61618982193066E-33,-1.03600583455278E-18,
-1.));
#7769=DIRECTION('ref_axis',(1.,0.,0.));
#7770=DIRECTION('',(0.,0.,-1.));
#7771=DIRECTION('center_axis',(-9.61618982193066E-33,1.03600583455278E-18,
1.));
#7772=DIRECTION('ref_axis',(1.,0.,0.));
#7773=DIRECTION('center_axis',(0.,0.,-1.));
#7774=DIRECTION('ref_axis',(1.,0.,0.));
#7775=DIRECTION('center_axis',(9.61618982193066E-33,-1.03600583455278E-18,
-1.));
#7776=DIRECTION('ref_axis',(1.,0.,0.));
#7777=DIRECTION('',(0.,0.,-1.));
#7778=DIRECTION('center_axis',(0.,0.,-1.));
#7779=DIRECTION('ref_axis',(1.,0.,0.));
#7780=DIRECTION('center_axis',(9.61618982193066E-33,-1.03600583455278E-18,
-1.));
#7781=DIRECTION('ref_axis',(1.,0.,0.));
#7782=DIRECTION('',(0.,0.,-1.));
#7783=DIRECTION('center_axis',(0.,0.,-1.));
#7784=DIRECTION('ref_axis',(1.,0.,0.));
#7785=DIRECTION('center_axis',(9.61618982193066E-33,-1.03600583455278E-18,
-1.));
#7786=DIRECTION('ref_axis',(1.,0.,0.));
#7787=DIRECTION('',(0.,0.,-1.));
#7788=DIRECTION('center_axis',(-9.61618982193066E-33,1.03600583455278E-18,
1.));
#7789=DIRECTION('ref_axis',(1.,0.,0.));
#7790=DIRECTION('center_axis',(0.,0.,-1.));
#7791=DIRECTION('ref_axis',(1.,0.,0.));
#7792=DIRECTION('center_axis',(9.61618982193066E-33,-1.03600583455278E-18,
-1.));
#7793=DIRECTION('ref_axis',(1.,0.,0.));
#7794=DIRECTION('',(0.,0.,-1.));
#7795=DIRECTION('center_axis',(0.,0.,-1.));
#7796=DIRECTION('ref_axis',(1.,0.,0.));
#7797=DIRECTION('center_axis',(0.,0.,-1.));
#7798=DIRECTION('ref_axis',(1.,0.,0.));
#7799=DIRECTION('center_axis',(0.,0.,1.));
#7800=DIRECTION('ref_axis',(1.,0.,0.));
#7801=DIRECTION('center_axis',(0.,0.,-1.));
#7802=DIRECTION('ref_axis',(1.,0.,0.));
#7803=DIRECTION('center_axis',(9.61618982193066E-33,-1.03600583455278E-18,
-1.));
#7804=DIRECTION('ref_axis',(1.,0.,0.));
#7805=DIRECTION('',(0.,0.,-1.));
#7806=DIRECTION('center_axis',(0.,0.,-1.));
#7807=DIRECTION('ref_axis',(1.,0.,0.));
#7808=DIRECTION('center_axis',(0.,0.,-1.));
#7809=DIRECTION('ref_axis',(1.,0.,0.));
#7810=DIRECTION('center_axis',(0.,0.,1.));
#7811=DIRECTION('ref_axis',(1.,0.,0.));
#7812=DIRECTION('center_axis',(0.,0.,-1.));
#7813=DIRECTION('ref_axis',(1.,0.,0.));
#7814=DIRECTION('',(0.,0.,-1.));
#7815=DIRECTION('center_axis',(0.,0.,1.));
#7816=DIRECTION('ref_axis',(1.,0.,0.));
#7817=DIRECTION('center_axis',(0.,0.,-1.));
#7818=DIRECTION('ref_axis',(1.,0.,0.));
#7819=DIRECTION('',(0.,0.,-1.));
#7820=DIRECTION('center_axis',(0.,0.,1.));
#7821=DIRECTION('ref_axis',(1.,0.,0.));
#7822=DIRECTION('center_axis',(0.,-1.,0.));
#7823=DIRECTION('ref_axis',(-1.,0.,0.));
#7824=DIRECTION('',(0.0523359562429438,0.,0.998629534754574));
#7825=DIRECTION('',(1.,0.,0.));
#7826=DIRECTION('',(-0.0523359562429438,0.,-0.998629534754574));
#7827=DIRECTION('',(1.,0.,0.));
#7828=DIRECTION('center_axis',(0.,-1.,0.));
#7829=DIRECTION('ref_axis',(-1.,0.,0.));
#7830=DIRECTION('',(0.,0.,-1.));
#7831=DIRECTION('',(1.,0.,0.));
#7832=DIRECTION('',(0.,0.,1.));
#7833=DIRECTION('',(1.,0.,0.));
#7834=DIRECTION('center_axis',(0.,-1.,0.));
#7835=DIRECTION('ref_axis',(-1.,0.,0.));
#7836=DIRECTION('',(0.,0.,-1.));
#7837=DIRECTION('',(1.,0.,0.));
#7838=DIRECTION('',(0.,0.,1.));
#7839=DIRECTION('',(1.,0.,0.));
#7840=DIRECTION('center_axis',(0.,-1.,0.));
#7841=DIRECTION('ref_axis',(-1.,0.,0.));
#7842=DIRECTION('',(0.,0.,-1.));
#7843=DIRECTION('',(1.,0.,0.));
#7844=DIRECTION('',(0.,0.,1.));
#7845=DIRECTION('',(1.,0.,0.));
#7846=DIRECTION('center_axis',(0.,1.,0.));
#7847=DIRECTION('ref_axis',(1.,0.,0.));
#7848=DIRECTION('',(-0.0523359562429438,0.,-0.998629534754574));
#7849=DIRECTION('',(-1.,0.,0.));
#7850=DIRECTION('',(0.0523359562429438,0.,0.998629534754574));
#7851=DIRECTION('',(-1.,0.,0.));
#7852=DIRECTION('center_axis',(0.,1.,0.));
#7853=DIRECTION('ref_axis',(1.,0.,0.));
#7854=DIRECTION('',(0.,0.,1.));
#7855=DIRECTION('',(-1.,0.,0.));
#7856=DIRECTION('',(0.,0.,-1.));
#7857=DIRECTION('',(-1.,0.,0.));
#7858=DIRECTION('center_axis',(0.,1.,0.));
#7859=DIRECTION('ref_axis',(1.,0.,0.));
#7860=DIRECTION('',(0.,0.,1.));
#7861=DIRECTION('',(-1.,0.,0.));
#7862=DIRECTION('',(0.,0.,-1.));
#7863=DIRECTION('',(-1.,0.,0.));
#7864=DIRECTION('center_axis',(0.,0.,1.));
#7865=DIRECTION('ref_axis',(1.,0.,0.));
#7866=DIRECTION('center_axis',(0.,0.,1.));
#7867=DIRECTION('ref_axis',(1.,0.,0.));
#7868=DIRECTION('center_axis',(0.,0.,1.));
#7869=DIRECTION('ref_axis',(1.,0.,0.));
#7870=DIRECTION('center_axis',(0.,0.,1.));
#7871=DIRECTION('ref_axis',(1.,0.,0.));
#7872=DIRECTION('center_axis',(0.,0.,1.));
#7873=DIRECTION('ref_axis',(1.,0.,0.));
#7874=DIRECTION('',(0.,1.,0.));
#7875=DIRECTION('',(0.,-1.,0.));
#7876=DIRECTION('center_axis',(0.,0.,1.));
#7877=DIRECTION('ref_axis',(1.,0.,0.));
#7878=DIRECTION('',(0.,-1.,0.));
#7879=DIRECTION('',(0.,1.,0.));
#7880=DIRECTION('center_axis',(0.,0.,1.));
#7881=DIRECTION('ref_axis',(1.,0.,0.));
#7882=DIRECTION('',(0.,-1.,0.));
#7883=DIRECTION('',(0.,1.,0.));
#7884=DIRECTION('center_axis',(0.,0.,1.));
#7885=DIRECTION('ref_axis',(1.,0.,0.));
#7886=DIRECTION('',(0.,-1.,0.));
#7887=DIRECTION('',(-1.,0.,0.));
#7888=DIRECTION('',(0.,1.,0.));
#7889=DIRECTION('center_axis',(0.,1.,0.));
#7890=DIRECTION('ref_axis',(1.,0.,0.));
#7891=DIRECTION('',(0.,0.,1.));
#7892=DIRECTION('',(-1.,0.,0.));
#7893=DIRECTION('',(0.,0.,-1.));
#7894=DIRECTION('center_axis',(-1.,0.,0.));
#7895=DIRECTION('ref_axis',(0.,-1.,0.));
#7896=DIRECTION('',(0.,-1.,0.));
#7897=DIRECTION('',(0.,-1.,1.03600583455278E-18));
#7898=DIRECTION('center_axis',(1.,0.,0.));
#7899=DIRECTION('ref_axis',(0.,1.,0.));
#7900=DIRECTION('',(0.,1.,0.));
#7901=DIRECTION('',(0.,1.,-1.03600583455278E-18));
#7902=DIRECTION('',(0.,1.,0.));
#7903=DIRECTION('center_axis',(1.,0.,0.));
#7904=DIRECTION('ref_axis',(0.,1.,0.));
#7905=DIRECTION('',(0.,1.,0.));
#7906=DIRECTION('',(0.,1.,-1.03600583455278E-18));
#7907=DIRECTION('',(0.,1.,0.));
#7908=DIRECTION('center_axis',(1.,0.,0.));
#7909=DIRECTION('ref_axis',(0.,1.,0.));
#7910=DIRECTION('',(0.,1.,0.));
#7911=DIRECTION('',(0.,1.,0.));
#7912=DIRECTION('center_axis',(0.998629534754574,0.,-0.0523359562429438));
#7913=DIRECTION('ref_axis',(-0.0523359562429438,0.,-0.998629534754574));
#7914=DIRECTION('',(0.,-1.,0.));
#7915=DIRECTION('',(5.42947651131849E-20,-1.,1.03600583455278E-18));
#7916=DIRECTION('',(0.,-1.,0.));
#7917=DIRECTION('center_axis',(0.,0.,1.));
#7918=DIRECTION('ref_axis',(1.,0.,0.));
#7919=DIRECTION('',(0.,-1.,0.));
#7920=DIRECTION('',(0.,-1.,0.));
#7921=DIRECTION('',(0.,-1.,0.));
#7922=DIRECTION('',(0.,1.,0.));
#7923=DIRECTION('',(0.,-1.,0.));
#7924=DIRECTION('',(0.,1.,0.));
#7925=DIRECTION('',(0.,-1.,0.));
#7926=DIRECTION('',(0.,-1.,0.));
#7927=DIRECTION('',(0.,-1.,0.));
#7928=DIRECTION('',(0.,1.,0.));
#7929=DIRECTION('',(0.,1.,0.));
#7930=DIRECTION('center_axis',(0.,0.,1.));
#7931=DIRECTION('ref_axis',(1.,0.,0.));
#7932=DIRECTION('center_axis',(-9.61618982193066E-33,1.03600583455278E-18,
1.));
#7933=DIRECTION('ref_axis',(1.,0.,0.));
#7934=DIRECTION('',(0.,0.,-1.));
#7935=DIRECTION('center_axis',(0.,0.,1.));
#7936=DIRECTION('ref_axis',(1.,0.,0.));
#7937=DIRECTION('',(0.,0.,-1.));
#7938=DIRECTION('center_axis',(1.,0.,0.));
#7939=DIRECTION('ref_axis',(0.,1.,0.));
#7940=DIRECTION('',(0.,1.,-1.03600583455278E-18));
#7941=DIRECTION('center_axis',(0.994044372876412,-0.108976074221552,-1.1933167131821E-14));
#7942=DIRECTION('ref_axis',(-0.108857570442347,-0.992963419871597,0.0466226999892957));
#7943=DIRECTION('center_axis',(-9.61618982193066E-33,1.03600583455278E-18,
1.));
#7944=DIRECTION('ref_axis',(1.,0.,9.61618982193066E-33));
#7945=DIRECTION('center_axis',(-9.61618982193066E-33,1.03600583455278E-18,
1.));
#7946=DIRECTION('ref_axis',(1.,0.,9.61618982193066E-33));
#7947=DIRECTION('',(-5.42947651131849E-20,-1.,1.03600583455278E-18));
#7948=DIRECTION('center_axis',(-1.,0.,0.));
#7949=DIRECTION('ref_axis',(0.,-1.,0.));
#7950=DIRECTION('',(0.,-1.,1.03600583455278E-18));
#7951=DIRECTION('center_axis',(-9.61618982193066E-33,1.03600583455278E-18,
1.));
#7952=DIRECTION('ref_axis',(1.,0.,9.61618982193066E-33));
#7953=DIRECTION('center_axis',(-1.,0.,0.));
#7954=DIRECTION('ref_axis',(0.,-1.,0.));
#7955=DIRECTION('center_axis',(-1.,0.,0.));
#7956=DIRECTION('ref_axis',(0.,-1.,0.));
#7957=DIRECTION('',(0.,-1.,1.03600583455278E-18));
#7958=DIRECTION('center_axis',(-0.999738255753194,0.0228783737088345,0.));
#7959=DIRECTION('ref_axis',(0.,0.,1.));
#7960=DIRECTION('center_axis',(-9.61618982193066E-33,1.03600583455278E-18,
1.));
#7961=DIRECTION('ref_axis',(1.,0.,9.61618982193066E-33));
#7962=DIRECTION('',(-5.42947651131849E-20,1.,-1.03600583455278E-18));
#7963=DIRECTION('center_axis',(-0.999738255790058,-0.0228783720979604,1.69987959829136E-9));
#7964=DIRECTION('ref_axis',(-0.022845652001536,0.998308458201847,0.0534630570326489));
#7965=DIRECTION('center_axis',(-0.375013085256251,-0.833398400631247,0.405970801550885));
#7966=DIRECTION('ref_axis',(-0.565498005067694,0.552672693214782,0.612180447612612));
#7967=DIRECTION('center_axis',(-7.78474640228738E-11,1.,0.));
#7968=DIRECTION('ref_axis',(0.,0.,1.));
#7969=DIRECTION('center_axis',(0.0522645732252412,-0.0522112666801462,0.997267465636596));
#7970=DIRECTION('ref_axis',(-0.998629534754574,0.,0.0523359562429445));
#7971=DIRECTION('center_axis',(0.361627795167438,-0.818371417997736,0.44664701943113));
#7972=DIRECTION('ref_axis',(0.514966362801186,0.574689674697898,0.636035708886648));
#7973=DIRECTION('center_axis',(0.994044372876412,0.108976074221546,-5.96658356591051E-15));
#7974=DIRECTION('ref_axis',(5.9211894646675E-15,7.40148683083438E-16,1.));
#7975=DIRECTION('center_axis',(-0.052263633556273,-0.0525535553916586,0.997249535684621));
#7976=DIRECTION('ref_axis',(-0.108857570442347,0.992963419871597,0.0466226999892949));
#7977=DIRECTION('center_axis',(0.,1.,0.));
#7978=DIRECTION('ref_axis',(0.998629534754574,0.,0.0523359562429438));
#7979=DIRECTION('center_axis',(0.375013085403515,-0.833398400816333,-0.405970801034895));
#7980=DIRECTION('ref_axis',(-0.565498005700927,-0.552672692935682,0.612180447279637));
#7981=DIRECTION('center_axis',(0.0522645732252408,0.0522112666801459,0.997267465636596));
#7982=DIRECTION('ref_axis',(-0.0228456520015352,-0.998308458201847,0.0534630570326489));
#7983=DIRECTION('center_axis',(-4.07418268117644E-12,-1.,-7.77400366303027E-11));
#7984=DIRECTION('ref_axis',(-0.998629534754574,0.,0.0523359562429438));
#7985=DIRECTION('center_axis',(-5.42947651131849E-20,1.,-1.03600583455278E-18));
#7986=DIRECTION('ref_axis',(-0.688354575693754,0.,0.725374371012288));
#7987=DIRECTION('center_axis',(-0.361627795167436,-0.818371417997736,-0.446647019431131));
#7988=DIRECTION('ref_axis',(0.514966362801185,-0.574689674697896,0.636035708886651));
#7989=DIRECTION('center_axis',(-0.0522636335562752,0.0525535553916633,0.99724953568462));
#7990=DIRECTION('ref_axis',(0.998629534754574,0.,0.0523359562429442));
#7991=DIRECTION('center_axis',(0.,-1.,0.));
#7992=DIRECTION('ref_axis',(0.,0.,1.));
#7993=DIRECTION('center_axis',(-5.42947651131849E-20,-1.,1.03600583455278E-18));
#7994=DIRECTION('ref_axis',(0.688354575693754,0.,0.725374371012288));
#7995=DIRECTION('',(5.42947651131849E-20,1.,-1.03600583455278E-18));
#7996=DIRECTION('center_axis',(-0.998629534754574,0.,-0.0523359562429438));
#7997=DIRECTION('ref_axis',(-0.0523359562429438,0.,0.998629534754574));
#7998=DIRECTION('center_axis',(-0.375013085256251,-0.833398400631247,0.405970801550885));
#7999=DIRECTION('ref_axis',(-0.565498005067695,0.552672693214781,0.612180447612612));
#8000=DIRECTION('center_axis',(-7.78474640228738E-11,1.,0.));
#8001=DIRECTION('ref_axis',(0.,0.,1.));
#8002=DIRECTION('center_axis',(-0.999738255790058,-0.0228783720979604,1.69987959829136E-9));
#8003=DIRECTION('ref_axis',(-0.022845652001536,0.998308458201847,0.0534630570326489));
#8004=DIRECTION('center_axis',(0.0522645732252412,-0.0522112666801462,0.997267465636596));
#8005=DIRECTION('ref_axis',(-0.998629534754574,0.,0.0523359562429445));
#8006=DIRECTION('center_axis',(0.361627795167442,-0.818371417997735,0.446647019431129));
#8007=DIRECTION('ref_axis',(0.514966362801186,0.574689674697898,0.636035708886649));
#8008=DIRECTION('center_axis',(0.994044372876412,0.108976074221546,-5.96658356591051E-15));
#8009=DIRECTION('ref_axis',(5.9211894646675E-15,7.40148683083438E-16,1.));
#8010=DIRECTION('center_axis',(0.,1.,0.));
#8011=DIRECTION('ref_axis',(0.998629534754574,0.,0.0523359562429438));
#8012=DIRECTION('center_axis',(-0.052263633556273,-0.0525535553916586,0.997249535684621));
#8013=DIRECTION('ref_axis',(-0.108857570442347,0.992963419871597,0.0466226999892949));
#8014=DIRECTION('center_axis',(0.375013085403515,-0.833398400816333,-0.405970801034895));
#8015=DIRECTION('ref_axis',(-0.565498005700926,-0.552672692935682,0.612180447279637));
#8016=DIRECTION('center_axis',(-0.999738255753194,0.0228783737088345,0.));
#8017=DIRECTION('ref_axis',(0.,0.,1.));
#8018=DIRECTION('center_axis',(-4.07418268117644E-12,-1.,-7.77400366303027E-11));
#8019=DIRECTION('ref_axis',(-0.998629534754574,0.,0.0523359562429438));
#8020=DIRECTION('center_axis',(0.0522645732252408,0.0522112666801459,0.997267465636596));
#8021=DIRECTION('ref_axis',(-0.0228456520015352,-0.998308458201847,0.0534630570326489));
#8022=DIRECTION('center_axis',(-5.42947651131849E-20,1.,-1.03600583455278E-18));
#8023=DIRECTION('ref_axis',(-0.688354575693754,0.,0.725374371012288));
#8024=DIRECTION('',(5.42947651131849E-20,-1.,1.03600583455278E-18));
#8025=DIRECTION('',(-5.42947651131849E-20,1.,-1.03600583455278E-18));
#8026=DIRECTION('center_axis',(-0.361627795167436,-0.818371417997736,-0.446647019431131));
#8027=DIRECTION('ref_axis',(0.51496636280118,-0.574689674697898,0.636035708886653));
#8028=DIRECTION('center_axis',(-0.0522636335562752,0.0525535553916633,0.99724953568462));
#8029=DIRECTION('ref_axis',(0.998629534754574,0.,0.0523359562429441));
#8030=DIRECTION('center_axis',(0.,-1.,0.));
#8031=DIRECTION('ref_axis',(0.,0.,1.));
#8032=DIRECTION('center_axis',(0.994044372876412,-0.108976074221552,-1.1933167131821E-14));
#8033=DIRECTION('ref_axis',(-0.108857570442347,-0.992963419871597,0.0466226999892957));
#8034=DIRECTION('center_axis',(-5.42947651131849E-20,-1.,1.03600583455278E-18));
#8035=DIRECTION('ref_axis',(0.688354575693754,0.,0.725374371012288));
#8036=DIRECTION('',(5.42947651131849E-20,1.,-1.03600583455278E-18));
#8037=DIRECTION('',(-5.42947651131849E-20,-1.,1.03600583455278E-18));
#8038=DIRECTION('center_axis',(0.998629534754574,0.,-0.0523359562429438));
#8039=DIRECTION('ref_axis',(-0.0523359562429438,0.,-0.998629534754574));
#8040=DIRECTION('center_axis',(-9.61618982193066E-33,1.03600583455278E-18,
1.));
#8041=DIRECTION('ref_axis',(1.,0.,9.61618982193066E-33));
#8042=DIRECTION('center_axis',(-0.998629534754574,0.,-0.0523359562429438));
#8043=DIRECTION('ref_axis',(-0.0523359562429438,0.,0.998629534754574));
#9193=CARTESIAN_POINT('',(0.,0.,0.));
#9194=CARTESIAN_POINT('Origin',(6.87409734069396,-2.22251806091942E-16,
0.7));
#9195=CARTESIAN_POINT('',(3.31825992066485,1.2493322588334,0.7));
#9196=CARTESIAN_POINT('',(4.3,1.27917501057225,0.7));
#9197=CARTESIAN_POINT('Ctrl Pts',(3.31826243508713,1.24933270901874,0.7));
#9198=CARTESIAN_POINT('Ctrl Pts',(3.64552542112514,1.25866821321074,0.7));
#9199=CARTESIAN_POINT('Ctrl Pts',(3.97277304530853,1.26856018917077,0.7));
#9200=CARTESIAN_POINT('Ctrl Pts',(4.30000000005992,1.27917501058303,0.7));
#9201=CARTESIAN_POINT('',(4.3,-1.27917501057184,0.7));
#9202=CARTESIAN_POINT('',(4.3,0.742407407407408,0.7));
#9203=CARTESIAN_POINT('',(3.31825992075695,-1.24933225883136,0.7));
#9204=CARTESIAN_POINT('Ctrl Pts',(4.3000000000599,-1.27917501058303,0.7));
#9205=CARTESIAN_POINT('Ctrl Pts',(3.97277304533917,-1.26856018917177,0.7));
#9206=CARTESIAN_POINT('Ctrl Pts',(3.64552542118644,-1.25866821321259,0.7));
#9207=CARTESIAN_POINT('Ctrl Pts',(3.3182624351791,-1.24933270902137,0.7));
#9208=CARTESIAN_POINT('',(3.26759951430388,-1.24789152572578,0.7));
#9209=CARTESIAN_POINT('Ctrl Pts',(3.26760216044043,-1.24789199949781,0.7));
#9210=CARTESIAN_POINT('Ctrl Pts',(3.27154046708102,-1.24840675231115,0.699999999449966));
#9211=CARTESIAN_POINT('Ctrl Pts',(3.27549053112987,-1.2488275353013,0.699997549264952));
#9212=CARTESIAN_POINT('Ctrl Pts',(3.27944900419773,-1.24915404112413,0.699995443099811));
#9213=CARTESIAN_POINT('Ctrl Pts',(3.28202272903949,-1.24936632907779,0.699994073710794));
#9214=CARTESIAN_POINT('Ctrl Pts',(3.28459959180148,-1.24953872742098,0.699992815093061));
#9215=CARTESIAN_POINT('Ctrl Pts',(3.28717866899733,-1.24967118132558,0.699992046536556));
#9216=CARTESIAN_POINT('Ctrl Pts',(3.28888409507617,-1.24975876704947,0.699991538325205));
#9217=CARTESIAN_POINT('Ctrl Pts',(3.29059037034979,-1.2498288805585,0.699991238158591));
#9218=CARTESIAN_POINT('Ctrl Pts',(3.29229723346923,-1.24988151179005,0.69999118215758));
#9219=CARTESIAN_POINT('Ctrl Pts',(3.29393274317941,-1.24993194283473,0.699991128497625));
#9220=CARTESIAN_POINT('Ctrl Pts',(3.29556870469678,-1.24996631998408,0.699991298652463));
#9221=CARTESIAN_POINT('Ctrl Pts',(3.29720488848534,-1.24998463806557,0.699991673963628));
#9222=CARTESIAN_POINT('Ctrl Pts',(3.29943508678369,-1.25000960650399,0.699992185531049));
#9223=CARTESIAN_POINT('Ctrl Pts',(3.30166551218918,-1.25000473681137,0.699993084765318));
#9224=CARTESIAN_POINT('Ctrl Pts',(3.30389557412726,-1.24997002667259,0.699994176731177));
#9225=CARTESIAN_POINT('Ctrl Pts',(3.30868977915254,-1.24989540653807,0.699996524248132));
#9226=CARTESIAN_POINT('Ctrl Pts',(3.31348068594496,-1.24968290539118,0.699999999312134));
#9227=CARTESIAN_POINT('Ctrl Pts',(3.3182624351791,-1.24933270902137,0.7));
#9228=CARTESIAN_POINT('',(1.1,-1.19266190204492,0.7));
#9229=CARTESIAN_POINT('Ctrl Pts',(3.26760216044045,-1.24789199949781,0.7));
#9230=CARTESIAN_POINT('Ctrl Pts',(2.54512260523322,-1.2274084473838,0.7));
#9231=CARTESIAN_POINT('Ctrl Pts',(1.82256951666701,-1.20959509718369,0.7));
#9232=CARTESIAN_POINT('Ctrl Pts',(1.09999999999999,-1.19266190204553,0.7));
#9233=CARTESIAN_POINT('',(1.1,1.19266190204492,0.7));
#9234=CARTESIAN_POINT('',(1.1,-0.696450594095222,0.7));
#9235=CARTESIAN_POINT('',(3.26759952419083,1.24789152650872,0.7));
#9236=CARTESIAN_POINT('Ctrl Pts',(1.09999999999999,1.19266190204553,0.7));
#9237=CARTESIAN_POINT('Ctrl Pts',(1.82256951996781,1.20959509726105,0.7));
#9238=CARTESIAN_POINT('Ctrl Pts',(2.54512261183467,1.22740844754655,0.7));
#9239=CARTESIAN_POINT('Ctrl Pts',(3.26760217034162,1.24789199977852,0.7));
#9240=CARTESIAN_POINT('Ctrl Pts',(3.3182624351791,1.24933270902137,0.7));
#9241=CARTESIAN_POINT('Ctrl Pts',(3.3143012451848,1.2496228108833,0.699999999430174));
#9242=CARTESIAN_POINT('Ctrl Pts',(3.31033365565543,1.24981842655856,0.699997549220164));
#9243=CARTESIAN_POINT('Ctrl Pts',(3.30636302717881,1.24991943948955,0.699995443052606));
#9244=CARTESIAN_POINT('Ctrl Pts',(3.30378139908369,1.24998511620097,0.699994073661998));
#9245=CARTESIAN_POINT('Ctrl Pts',(3.3011989045204,1.25001078941611,0.699992815050698));
#9246=CARTESIAN_POINT('Ctrl Pts',(3.29861646861803,1.2499964568765,0.699992046505716));
#9247=CARTESIAN_POINT('Ctrl Pts',(3.2969088217217,1.24998697942277,0.699991538302026));
#9248=CARTESIAN_POINT('Ctrl Pts',(3.29520131971864,1.24996000972381,0.699991238145114));
#9249=CARTESIAN_POINT('Ctrl Pts',(3.29349422410899,1.24991555258537,0.699991182154076));
#9250=CARTESIAN_POINT('Ctrl Pts',(3.29185849176351,1.24987295392896,0.699991128503682));
#9251=CARTESIAN_POINT('Ctrl Pts',(3.29022322047391,1.2498143016413,0.699991298668259));
#9252=CARTESIAN_POINT('Ctrl Pts',(3.28858863969825,1.2497396036024,0.699991673987721));
#9253=CARTESIAN_POINT('Ctrl Pts',(3.286360626573,1.24963778654105,0.699992185566407));
#9254=CARTESIAN_POINT('Ctrl Pts',(3.28413408201674,1.24950616665997,0.699993084809042));
#9255=CARTESIAN_POINT('Ctrl Pts',(3.2819095957713,1.24934477520901,0.699994176777649));
#9256=CARTESIAN_POINT('Ctrl Pts',(3.27712738077041,1.24899781481787,0.699996524298861));
#9257=CARTESIAN_POINT('Ctrl Pts',(3.27235629258357,1.24851338385513,0.699999999330822));
#9258=CARTESIAN_POINT('Ctrl Pts',(3.26760217026193,1.24789200078152,0.699999999999999));
#9259=CARTESIAN_POINT('',(3.15,1.,0.7));
#9260=CARTESIAN_POINT('Origin',(3.3,1.,0.7));
#9261=CARTESIAN_POINT('',(3.15,-1.,0.7));
#9262=CARTESIAN_POINT('Origin',(3.3,-1.,0.7));
#9263=CARTESIAN_POINT('',(1.6,-4.89858719658941E-17,0.7));
#9264=CARTESIAN_POINT('Origin',(2.,0.,0.7));
#9265=CARTESIAN_POINT('Origin',(9.9,-1.,0.8));
#9266=CARTESIAN_POINT('',(9.75,-1.,0.9));
#9267=CARTESIAN_POINT('Origin',(9.9,-1.,0.9));
#9268=CARTESIAN_POINT('',(9.75,-1.,0.7));
#9269=CARTESIAN_POINT('',(9.75,-1.,0.8));
#9270=CARTESIAN_POINT('Origin',(9.9,-1.,0.7));
#9271=CARTESIAN_POINT('Origin',(3.3,-1.,0.8));
#9272=CARTESIAN_POINT('',(3.15,-1.,0.9));
#9273=CARTESIAN_POINT('Origin',(3.3,-1.,0.9));
#9274=CARTESIAN_POINT('',(3.15,-1.,0.8));
#9275=CARTESIAN_POINT('Origin',(3.3,1.,0.8));
#9276=CARTESIAN_POINT('',(3.15,1.,0.9));
#9277=CARTESIAN_POINT('Origin',(3.3,1.,0.9));
#9278=CARTESIAN_POINT('',(3.15,1.,0.8));
#9279=CARTESIAN_POINT('Origin',(9.9,1.,0.8));
#9280=CARTESIAN_POINT('',(9.75,1.,0.9));
#9281=CARTESIAN_POINT('Origin',(9.9,1.,0.9));
#9282=CARTESIAN_POINT('',(9.75,1.,0.7));
#9283=CARTESIAN_POINT('',(9.75,1.,0.8));
#9284=CARTESIAN_POINT('Origin',(9.9,1.,0.7));
#9285=CARTESIAN_POINT('Origin',(2.,0.,0.75));
#9286=CARTESIAN_POINT('',(1.7,3.67394039744206E-17,0.9));
#9287=CARTESIAN_POINT('Origin',(2.,0.,0.9));
#9288=CARTESIAN_POINT('',(1.7,3.67394039744206E-17,0.6));
#9289=CARTESIAN_POINT('',(1.7,3.67394039744206E-17,0.75));
#9290=CARTESIAN_POINT('Origin',(2.,0.,0.6));
#9291=CARTESIAN_POINT('Origin',(2.,0.,0.6));
#9292=CARTESIAN_POINT('',(1.83,-2.0818995585505E-17,0.6));
#9293=CARTESIAN_POINT('Origin',(2.,0.,0.6));
#9294=CARTESIAN_POINT('Origin',(11.2,0.,0.75));
#9295=CARTESIAN_POINT('',(10.9,3.67394039744206E-17,0.9));
#9296=CARTESIAN_POINT('Origin',(11.2,0.,0.9));
#9297=CARTESIAN_POINT('',(10.9,3.67394039744206E-17,0.6));
#9298=CARTESIAN_POINT('',(10.9,3.67394039744206E-17,0.75));
#9299=CARTESIAN_POINT('Origin',(11.2,0.,0.6));
#9300=CARTESIAN_POINT('Origin',(11.2,0.,0.6));
#9301=CARTESIAN_POINT('',(11.03,-2.0818995585505E-17,0.6));
#9302=CARTESIAN_POINT('Origin',(11.2,0.,0.6));
#9303=CARTESIAN_POINT('Origin',(2.,0.,0.45));
#9304=CARTESIAN_POINT('',(1.83,-2.0818995585505E-17,0.32));
#9305=CARTESIAN_POINT('',(1.83,2.0818995585505E-17,0.45));
#9306=CARTESIAN_POINT('Origin',(2.,0.,0.32));
#9307=CARTESIAN_POINT('Origin',(11.2,0.,0.45));
#9308=CARTESIAN_POINT('',(11.03,-2.0818995585505E-17,0.32));
#9309=CARTESIAN_POINT('',(11.03,2.0818995585505E-17,0.45));
#9310=CARTESIAN_POINT('Origin',(11.2,0.,0.32));
#9311=CARTESIAN_POINT('Origin',(12.4,-0.72,0.32));
#9312=CARTESIAN_POINT('',(0.200274469199584,-0.72,0.));
#9313=CARTESIAN_POINT('',(0.217044958570157,-0.72,0.32));
#9314=CARTESIAN_POINT('',(0.225070308370679,-0.72,0.473132796510599));
#9315=CARTESIAN_POINT('',(0.,-0.72,0.));
#9316=CARTESIAN_POINT('',(9.63649764092939,-0.72,0.));
#9317=CARTESIAN_POINT('',(0.0167704893705732,-0.72,0.32));
#9318=CARTESIAN_POINT('',(0.0253444014197637,-0.72,0.483599987759188));
#9319=CARTESIAN_POINT('',(-0.1,-0.72,0.32));
#9320=CARTESIAN_POINT('Origin',(12.4,-0.72,0.32));
#9321=CARTESIAN_POINT('',(0.9,-0.72,0.32));
#9322=CARTESIAN_POINT('',(0.9,-0.72,0.));
#9323=CARTESIAN_POINT('',(0.9,-0.72,0.16));
#9324=CARTESIAN_POINT('',(1.1,-0.72,0.32));
#9325=CARTESIAN_POINT('',(-0.1,-0.72,0.32));
#9326=CARTESIAN_POINT('',(1.1,-0.72,0.));
#9327=CARTESIAN_POINT('',(1.1,-0.72,0.16));
#9328=CARTESIAN_POINT('',(9.63649764092939,-0.72,0.));
#9329=CARTESIAN_POINT('Origin',(12.4,-0.72,0.32));
#9330=CARTESIAN_POINT('',(4.3,-0.72,0.32));
#9331=CARTESIAN_POINT('',(4.3,-0.72,0.));
#9332=CARTESIAN_POINT('',(4.3,-0.72,0.16));
#9333=CARTESIAN_POINT('',(4.5,-0.72,0.32));
#9334=CARTESIAN_POINT('',(-0.1,-0.72,0.32));
#9335=CARTESIAN_POINT('',(4.5,-0.72,0.));
#9336=CARTESIAN_POINT('',(4.5,-0.72,0.16));
#9337=CARTESIAN_POINT('',(9.63649764092939,-0.72,0.));
#9338=CARTESIAN_POINT('Origin',(12.4,-0.72,0.32));
#9339=CARTESIAN_POINT('',(8.7,-0.72,0.32));
#9340=CARTESIAN_POINT('',(8.7,-0.72,0.));
#9341=CARTESIAN_POINT('',(8.7,-0.72,0.16));
#9342=CARTESIAN_POINT('',(8.9,-0.72,0.32));
#9343=CARTESIAN_POINT('',(-0.1,-0.72,0.32));
#9344=CARTESIAN_POINT('',(8.9,-0.72,0.));
#9345=CARTESIAN_POINT('',(8.9,-0.72,0.16));
#9346=CARTESIAN_POINT('',(9.63649764092939,-0.72,0.));
#9347=CARTESIAN_POINT('Origin',(-0.0999999999999996,0.72,0.32));
#9348=CARTESIAN_POINT('',(0.217044958570158,0.72,0.32));
#9349=CARTESIAN_POINT('',(0.200274469199584,0.72,0.));
#9350=CARTESIAN_POINT('',(0.207951231396534,0.72,0.146481348799182));
#9351=CARTESIAN_POINT('',(0.0167704893705736,0.72,0.32));
#9352=CARTESIAN_POINT('',(12.4,0.72,0.32));
#9353=CARTESIAN_POINT('',(0.,0.72,0.));
#9354=CARTESIAN_POINT('',(0.00822532444561912,0.72,0.156948540047771));
#9355=CARTESIAN_POINT('',(3.38649764092939,0.72,0.));
#9356=CARTESIAN_POINT('Origin',(-0.0999999999999996,0.72,0.32));
#9357=CARTESIAN_POINT('',(0.9,0.72,0.));
#9358=CARTESIAN_POINT('',(0.9,0.72,0.32));
#9359=CARTESIAN_POINT('',(0.9,0.72,0.16));
#9360=CARTESIAN_POINT('',(1.1,0.72,0.));
#9361=CARTESIAN_POINT('',(3.38649764092939,0.72,0.));
#9362=CARTESIAN_POINT('',(1.1,0.72,0.32));
#9363=CARTESIAN_POINT('',(1.1,0.72,0.16));
#9364=CARTESIAN_POINT('',(12.4,0.72,0.32));
#9365=CARTESIAN_POINT('Origin',(-0.0999999999999996,0.72,0.32));
#9366=CARTESIAN_POINT('',(4.3,0.72,0.));
#9367=CARTESIAN_POINT('',(4.3,0.72,0.32));
#9368=CARTESIAN_POINT('',(4.3,0.72,0.16));
#9369=CARTESIAN_POINT('',(4.5,0.72,0.));
#9370=CARTESIAN_POINT('',(3.38649764092939,0.72,0.));
#9371=CARTESIAN_POINT('',(4.5,0.72,0.32));
#9372=CARTESIAN_POINT('',(4.5,0.72,0.16));
#9373=CARTESIAN_POINT('',(12.4,0.72,0.32));
#9374=CARTESIAN_POINT('Origin',(6.15,0.,0.32));
#9375=CARTESIAN_POINT('',(1.6,-4.89858719658941E-17,0.32));
#9376=CARTESIAN_POINT('Origin',(2.,0.,0.32));
#9377=CARTESIAN_POINT('Origin',(6.15,0.,0.32));
#9378=CARTESIAN_POINT('',(10.8,-4.89858719658942E-17,0.32));
#9379=CARTESIAN_POINT('Origin',(11.2,0.,0.32));
#9380=CARTESIAN_POINT('Origin',(6.15,0.,0.32));
#9381=CARTESIAN_POINT('',(0.217044958570157,-0.75,0.32));
#9382=CARTESIAN_POINT('',(0.0167704893705736,-0.75,0.32));
#9383=CARTESIAN_POINT('Origin',(6.15,0.,0.32));
#9384=CARTESIAN_POINT('',(0.9,0.696450594095222,0.32));
#9385=CARTESIAN_POINT('',(1.1,-0.696450594095222,0.32));
#9386=CARTESIAN_POINT('Origin',(6.15,0.,0.32));
#9387=CARTESIAN_POINT('',(4.3,0.742407407407408,0.32));
#9388=CARTESIAN_POINT('',(4.5,-0.742407407407408,0.32));
#9389=CARTESIAN_POINT('Origin',(6.15,0.,0.32));
#9390=CARTESIAN_POINT('',(8.7,0.72,0.32));
#9391=CARTESIAN_POINT('',(8.7,0.844259259259259,0.32));
#9392=CARTESIAN_POINT('',(8.9,0.72,0.32));
#9393=CARTESIAN_POINT('',(12.4,0.72,0.32));
#9394=CARTESIAN_POINT('',(8.9,-0.844259259259259,0.32));
#9395=CARTESIAN_POINT('Origin',(-0.0999999999999996,0.72,0.32));
#9396=CARTESIAN_POINT('',(8.7,0.72,0.));
#9397=CARTESIAN_POINT('',(8.7,0.72,0.16));
#9398=CARTESIAN_POINT('',(8.9,0.72,0.));
#9399=CARTESIAN_POINT('',(3.38649764092939,0.72,0.));
#9400=CARTESIAN_POINT('',(8.9,0.72,0.16));
#9401=CARTESIAN_POINT('Origin',(12.4,1.99376954809806,0.));
#9402=CARTESIAN_POINT('',(12.4,1.91212902562343,0.));
#9403=CARTESIAN_POINT('',(12.4,-1.91212902562343,0.));
#9404=CARTESIAN_POINT('',(12.4,1.99376954809806,0.));
#9405=CARTESIAN_POINT('',(12.4,-1.8833055216247,0.604732563714112));
#9406=CARTESIAN_POINT('Ctrl Pts',(12.4,-1.8833055216247,0.604732563714112));
#9407=CARTESIAN_POINT('Ctrl Pts',(12.4,-1.88809880980762,0.504101072758768));
#9408=CARTESIAN_POINT('Ctrl Pts',(12.4,-1.89289370245628,0.403468941627095));
#9409=CARTESIAN_POINT('Ctrl Pts',(12.4,-1.90250151416087,0.201891903194028));
#9410=CARTESIAN_POINT('Ctrl Pts',(12.4,-1.90731451170285,0.100945553925438));
#9411=CARTESIAN_POINT('Ctrl Pts',(12.4,-1.91212902562343,0.));
#9412=CARTESIAN_POINT('',(12.4,-1.78288409287054,0.7));
#9413=CARTESIAN_POINT('Ctrl Pts',(12.4000000030461,-1.78288409409899,0.7));
#9414=CARTESIAN_POINT('Ctrl Pts',(12.4000000066823,-1.79082830277209,0.699999997040196));
#9415=CARTESIAN_POINT('Ctrl Pts',(12.4000021328137,-1.79871128857748,0.699006690321208));
#9416=CARTESIAN_POINT('Ctrl Pts',(12.4000039827682,-1.8063921320806,0.697119229445379));
#9417=CARTESIAN_POINT('Ctrl Pts',(12.4000049365067,-1.81035196808589,0.69614615460905));
#9418=CARTESIAN_POINT('Ctrl Pts',(12.4000058167808,-1.81425808325963,0.694934510320783));
#9419=CARTESIAN_POINT('Ctrl Pts',(12.400006432968,-1.81808986884151,0.693492707237305));
#9420=CARTESIAN_POINT('Ctrl Pts',(12.4000076352846,-1.82556652433459,0.690679432664999));
#9421=CARTESIAN_POINT('Ctrl Pts',(12.4000076271954,-1.83268048852469,0.687023315130674));
#9422=CARTESIAN_POINT('Ctrl Pts',(12.4000063864816,-1.83928589538344,0.682605693351404));
#9423=CARTESIAN_POINT('Ctrl Pts',(12.4000055969106,-1.84348947395919,0.679794387301037));
#9424=CARTESIAN_POINT('Ctrl Pts',(12.400004329084,-1.84748689691167,0.676673627174617));
#9425=CARTESIAN_POINT('Ctrl Pts',(12.4000032503406,-1.8512341074341,0.673255429390325));
#9426=CARTESIAN_POINT('Ctrl Pts',(12.4000023796213,-1.85425870830395,0.670496394655072));
#9427=CARTESIAN_POINT('Ctrl Pts',(12.4000016297172,-1.85710218072175,0.667559826261508));
#9428=CARTESIAN_POINT('Ctrl Pts',(12.4000016274617,-1.859744520612,0.664455546516084));
#9429=CARTESIAN_POINT('Ctrl Pts',(12.4000016230979,-1.86485672743849,0.658449612092435));
#9430=CARTESIAN_POINT('Ctrl Pts',(12.4000041080363,-1.86921906069885,0.651817317967817));
#9431=CARTESIAN_POINT('Ctrl Pts',(12.40000495371,-1.8727702927896,0.64472299566344));
#9432=CARTESIAN_POINT('Ctrl Pts',(12.4000050555652,-1.8731980125259,0.643868536819953));
#9433=CARTESIAN_POINT('Ctrl Pts',(12.4000051394069,-1.87361391018412,0.643007349425002));
#9434=CARTESIAN_POINT('Ctrl Pts',(12.4000052029357,-1.87401783114888,0.642139703315781));
#9435=CARTESIAN_POINT('Ctrl Pts',(12.4000057294153,-1.87736522853405,0.634949295858174));
#9436=CARTESIAN_POINT('Ctrl Pts',(12.4000043880804,-1.87985460663586,0.627401584261416));
#9437=CARTESIAN_POINT('Ctrl Pts',(12.4000025112034,-1.88143175301701,0.619663949188762));
#9438=CARTESIAN_POINT('Ctrl Pts',(12.4000013193515,-1.88243327046239,0.614750406220363));
#9439=CARTESIAN_POINT('Ctrl Pts',(12.4,-1.88306607129604,0.609759643802656));
#9440=CARTESIAN_POINT('Ctrl Pts',(12.4,-1.8833055216247,0.604732563714112));
#9441=CARTESIAN_POINT('',(12.4,1.78288409287164,0.7));
#9442=CARTESIAN_POINT('',(12.4,0.99688477404903,0.7));
#9443=CARTESIAN_POINT('',(12.4,1.8833055216247,0.604732563714112));
#9444=CARTESIAN_POINT('Ctrl Pts',(12.4,1.8833055216247,0.604732563714112));
#9445=CARTESIAN_POINT('Ctrl Pts',(12.4,1.88292893537322,0.612638709665068));
#9446=CARTESIAN_POINT('Ctrl Pts',(12.4000029905988,1.88158186833012,0.620459457162159));
#9447=CARTESIAN_POINT('Ctrl Pts',(12.400004351969,1.87934739482834,0.62803467841275));
#9448=CARTESIAN_POINT('Ctrl Pts',(12.4000050124983,1.87826324073514,0.631710133556493));
#9449=CARTESIAN_POINT('Ctrl Pts',(12.4000053733669,1.87696936339782,0.63532777623417));
#9450=CARTESIAN_POINT('Ctrl Pts',(12.4000053391329,1.87547104796815,0.638868146717817));
#9451=CARTESIAN_POINT('Ctrl Pts',(12.4000052683671,1.872373843052,0.646186534188034));
#9452=CARTESIAN_POINT('Ctrl Pts',(12.4000032465668,1.86844110215533,0.653093304890266));
#9453=CARTESIAN_POINT('Ctrl Pts',(12.4000021327941,1.86374151467895,0.659427433016556));
#9454=CARTESIAN_POINT('Ctrl Pts',(12.4000018304335,1.86246569800928,0.66114698527342));
#9455=CARTESIAN_POINT('Ctrl Pts',(12.4000016226794,1.86113309763036,0.662824214875179));
#9456=CARTESIAN_POINT('Ctrl Pts',(12.400001625255,1.85974452038344,0.664455546516227));
#9457=CARTESIAN_POINT('Ctrl Pts',(12.4000016287814,1.85784336180007,0.666689070188443));
#9458=CARTESIAN_POINT('Ctrl Pts',(12.400002024929,1.85583728779192,0.668836587948716));
#9459=CARTESIAN_POINT('Ctrl Pts',(12.4000025639666,1.85373364862045,0.670894373083513));
#9460=CARTESIAN_POINT('Ctrl Pts',(12.400004021536,1.84804536272624,0.676458668669153));
#9461=CARTESIAN_POINT('Ctrl Pts',(12.4000062945443,1.84171268252251,0.681305055194542));
#9462=CARTESIAN_POINT('Ctrl Pts',(12.4000070319583,1.83490078417639,0.685381489016216));
#9463=CARTESIAN_POINT('Ctrl Pts',(12.4000075068619,1.8305138392177,0.688006761722114));
#9464=CARTESIAN_POINT('Ctrl Pts',(12.4000074483741,1.82592714021755,0.69031203082117));
#9465=CARTESIAN_POINT('Ctrl Pts',(12.4000068708525,1.82117863971551,0.692273867243687));
#9466=CARTESIAN_POINT('Ctrl Pts',(12.4000059767178,1.81382688138917,0.695311236040001));
#9467=CARTESIAN_POINT('Ctrl Pts',(12.4000038254996,1.80617119073902,0.697493343451155));
#9468=CARTESIAN_POINT('Ctrl Pts',(12.4000020685374,1.7983596509798,0.698751345219246));
#9469=CARTESIAN_POINT('Ctrl Pts',(12.4000009204513,1.79325520389048,0.699573385900268));
#9470=CARTESIAN_POINT('Ctrl Pts',(12.400000005426,1.78808359082883,0.699999998062804));
#9471=CARTESIAN_POINT('Ctrl Pts',(12.4000000030461,1.78288409409899,0.7));
#9472=CARTESIAN_POINT('Ctrl Pts',(12.4,1.91212902562343,0.));
#9473=CARTESIAN_POINT('Ctrl Pts',(12.4,1.90731404243129,0.1009553931071));
#9474=CARTESIAN_POINT('Ctrl Pts',(12.4,1.9025005759122,0.201911581737034));
#9475=CARTESIAN_POINT('Ctrl Pts',(12.4,1.89289276481806,0.403488620176902));
#9476=CARTESIAN_POINT('Ctrl Pts',(12.4,1.88809834114759,0.504110911924693));
#9477=CARTESIAN_POINT('Ctrl Pts',(12.4,1.8833055216247,0.604732563714112));
#9478=CARTESIAN_POINT('Origin',(8.9,-1.68851851851852,0.));
#9479=CARTESIAN_POINT('',(8.9,1.62420669932031,0.));
#9480=CARTESIAN_POINT('',(8.9,-1.68851851851852,0.));
#9481=CARTESIAN_POINT('',(8.9,1.59320117118329,0.605106081470792));
#9482=CARTESIAN_POINT('Ctrl Pts',(8.9,1.59320117118329,0.605106081470792));
#9483=CARTESIAN_POINT('Ctrl Pts',(8.9,1.59837103562161,0.504197738990529));
#9484=CARTESIAN_POINT('Ctrl Pts',(8.9,1.60354126123154,0.403288838380538));
#9485=CARTESIAN_POINT('Ctrl Pts',(8.9,1.61387642009944,0.201587196710533));
#9486=CARTESIAN_POINT('Ctrl Pts',(8.9,1.61904141157348,0.100793304842659));
#9487=CARTESIAN_POINT('Ctrl Pts',(8.9,1.62420669932031,0.));
#9488=CARTESIAN_POINT('',(8.9,1.49312521822106,0.7));
#9489=CARTESIAN_POINT('Ctrl Pts',(8.9,1.49312521822106,0.7));
#9490=CARTESIAN_POINT('Ctrl Pts',(8.9,1.50104136823484,0.7));
#9491=CARTESIAN_POINT('Ctrl Pts',(8.90000131173634,1.50889623314995,0.699007530025307));
#9492=CARTESIAN_POINT('Ctrl Pts',(8.90000245364087,1.51654949575132,0.697121675771258));
#9493=CARTESIAN_POINT('Ctrl Pts',(8.9000030153269,1.52031402289636,0.696194051841344));
#9494=CARTESIAN_POINT('Ctrl Pts',(8.90000353645954,1.52402976767023,0.695049421358208));
#9495=CARTESIAN_POINT('Ctrl Pts',(8.90000391188735,1.52767894577544,0.693695149285802));
#9496=CARTESIAN_POINT('Ctrl Pts',(8.90000468147812,1.53515940869299,0.690919022244083));
#9497=CARTESIAN_POINT('Ctrl Pts',(8.90000470661952,1.54227958804117,0.687295426711095));
#9498=CARTESIAN_POINT('Ctrl Pts',(8.9000039635008,1.54889410374269,0.682907715777054));
#9499=CARTESIAN_POINT('Ctrl Pts',(8.90000349228854,1.55308837416723,0.680125464281631));
#9500=CARTESIAN_POINT('Ctrl Pts',(8.90000272405863,1.55707914411963,0.677034908766328));
#9501=CARTESIAN_POINT('Ctrl Pts',(8.90000205379677,1.56082314136721,0.673648333128258));
#9502=CARTESIAN_POINT('Ctrl Pts',(8.90000149471997,1.56394607304962,0.670823532879853));
#9503=CARTESIAN_POINT('Ctrl Pts',(8.90000100172653,1.56687805273397,0.667809941545923));
#9504=CARTESIAN_POINT('Ctrl Pts',(8.90000100003,1.56959740049228,0.664618488856983));
#9505=CARTESIAN_POINT('Ctrl Pts',(8.90000099684156,1.57470809805256,0.658620525035968));
#9506=CARTESIAN_POINT('Ctrl Pts',(8.90000253934467,1.57907071782202,0.651995745956818));
#9507=CARTESIAN_POINT('Ctrl Pts',(8.90000305932469,1.58262507990443,0.644909256877938));
#9508=CARTESIAN_POINT('Ctrl Pts',(8.90000311559331,1.58300970826793,0.644142406277414));
#9509=CARTESIAN_POINT('Ctrl Pts',(8.9000031627798,1.58338482682255,0.643370127200485));
#9510=CARTESIAN_POINT('Ctrl Pts',(8.90000319981124,1.58375032531468,0.642592615892991));
#9511=CARTESIAN_POINT('Ctrl Pts',(8.90000354178946,1.58712563340961,0.635412448897651));
#9512=CARTESIAN_POINT('Ctrl Pts',(8.90000272882427,1.58964525157545,0.627871187463612));
#9513=CARTESIAN_POINT('Ctrl Pts',(8.90000156924769,1.59125549206429,0.620136848214628));
#9514=CARTESIAN_POINT('Ctrl Pts',(8.90000082792478,1.59228492658837,0.615192247765769));
#9515=CARTESIAN_POINT('Ctrl Pts',(8.89999999997262,1.59294182914154,0.610168076493048));
#9516=CARTESIAN_POINT('Ctrl Pts',(8.9000000009702,1.5932011715731,0.605106081469384));
#9517=CARTESIAN_POINT('',(8.9,-1.49312521822001,0.7));
#9518=CARTESIAN_POINT('',(8.9,-0.844259259259259,0.7));
#9519=CARTESIAN_POINT('',(8.9,-1.59320117118329,0.605106081470792));
#9520=CARTESIAN_POINT('Ctrl Pts',(8.90000000097019,-1.5932011715731,0.605106081469384));
#9521=CARTESIAN_POINT('Ctrl Pts',(8.89999999941083,-1.59279578158415,0.613018716877257));
#9522=CARTESIAN_POINT('Ctrl Pts',(8.90000185372291,-1.59142151714118,0.620841302874248));
#9523=CARTESIAN_POINT('Ctrl Pts',(8.90000269095591,-1.58916270068609,0.628413601005994));
#9524=CARTESIAN_POINT('Ctrl Pts',(8.90000316003867,-1.58789713677684,0.632656188846207));
#9525=CARTESIAN_POINT('Ctrl Pts',(8.90000337414869,-1.58635289833986,0.636820251299613));
#9526=CARTESIAN_POINT('Ctrl Pts',(8.90000326408749,-1.58453800492682,0.640875626603871));
#9527=CARTESIAN_POINT('Ctrl Pts',(8.9000030675631,-1.58129734600662,0.648116871770122));
#9528=CARTESIAN_POINT('Ctrl Pts',(8.90000169351568,-1.5772322800227,0.654932667693845));
#9529=CARTESIAN_POINT('Ctrl Pts',(8.90000116172667,-1.57240747726376,0.66116027211862));
#9530=CARTESIAN_POINT('Ctrl Pts',(8.90000106146602,-1.57149783490479,0.662334391157823));
#9531=CARTESIAN_POINT('Ctrl Pts',(8.90000099955281,-1.57056105641498,0.663487533005214));
#9532=CARTESIAN_POINT('Ctrl Pts',(8.90000100072893,-1.56959740053727,0.664618488856962));
#9533=CARTESIAN_POINT('Ctrl Pts',(8.9000010030487,-1.56769671285427,0.666849154291726));
#9534=CARTESIAN_POINT('Ctrl Pts',(8.90000124864079,-1.56569149899762,0.668993559652069));
#9535=CARTESIAN_POINT('Ctrl Pts',(8.90000158179872,-1.56358911460694,0.671047966011734));
#9536=CARTESIAN_POINT('Ctrl Pts',(8.90000248280001,-1.55790336961918,0.676603957919834));
#9537=CARTESIAN_POINT('Ctrl Pts',(8.90000387848177,-1.55157399841983,0.681441805123218));
#9538=CARTESIAN_POINT('Ctrl Pts',(8.90000432886686,-1.54476515293017,0.68550782533293));
#9539=CARTESIAN_POINT('Ctrl Pts',(8.9000046162921,-1.54041990676133,0.688102664467623));
#9540=CARTESIAN_POINT('Ctrl Pts',(8.90000458123012,-1.53587841548674,0.69038248607508));
#9541=CARTESIAN_POINT('Ctrl Pts',(8.90000422571091,-1.53117752164703,0.692323975790708));
#9542=CARTESIAN_POINT('Ctrl Pts',(8.90000367147839,-1.52384911813356,0.695350638493274));
#9543=CARTESIAN_POINT('Ctrl Pts',(8.9000023358238,-1.51621796414731,0.697522741667433));
#9544=CARTESIAN_POINT('Ctrl Pts',(8.90000125519218,-1.50843132129101,0.698770821080692));
#9545=CARTESIAN_POINT('Ctrl Pts',(8.90000055451733,-1.5033825102871,0.699580068042664));
#9546=CARTESIAN_POINT('Ctrl Pts',(8.9,-1.49826772866746,0.7));
#9547=CARTESIAN_POINT('Ctrl Pts',(8.9,-1.49312521822106,0.7));
#9548=CARTESIAN_POINT('',(8.9,-1.62420669932031,0.));
#9549=CARTESIAN_POINT('Ctrl Pts',(8.9,-1.62420669932031,0.));
#9550=CARTESIAN_POINT('Ctrl Pts',(8.9,-1.61904139377919,0.100793652073202));
#9551=CARTESIAN_POINT('Ctrl Pts',(8.9,-1.61387638451174,0.201587891198165));
#9552=CARTESIAN_POINT('Ctrl Pts',(8.9,-1.60354122564866,0.403289532862703));
#9553=CARTESIAN_POINT('Ctrl Pts',(8.9,-1.59837101783099,0.50419808623799));
#9554=CARTESIAN_POINT('Ctrl Pts',(8.9,-1.59320117118329,0.605106081470792));
#9555=CARTESIAN_POINT('',(8.9,-1.68851851851852,0.));
#9556=CARTESIAN_POINT('Origin',(4.5,-1.48481481481482,0.));
#9557=CARTESIAN_POINT('',(4.5,1.41772989878425,0.));
#9558=CARTESIAN_POINT('',(4.5,-1.48481481481482,0.));
#9559=CARTESIAN_POINT('',(4.5,1.38566996325095,0.605286533624017));
#9560=CARTESIAN_POINT('Ctrl Pts',(4.5,1.38566996325095,0.605286533624017));
#9561=CARTESIAN_POINT('Ctrl Pts',(4.5,1.3910232158183,0.504222354021684));
#9562=CARTESIAN_POINT('Ctrl Pts',(4.5,1.39637635187357,0.403158168247774));
#9563=CARTESIAN_POINT('Ctrl Pts',(4.5,1.4070629957395,0.201395990303158));
#9564=CARTESIAN_POINT('Ctrl Pts',(4.5,1.41239650438775,0.100697998177668));
#9565=CARTESIAN_POINT('Ctrl Pts',(4.5,1.41772989878425,0.));
#9566=CARTESIAN_POINT('',(4.5,1.28575421950843,0.7));
#9567=CARTESIAN_POINT('Ctrl Pts',(4.5,1.28575421950843,0.7));
#9568=CARTESIAN_POINT('Ctrl Pts',(4.5,1.29366545802379,0.7));
#9569=CARTESIAN_POINT('Ctrl Pts',(4.50000067540813,1.30151306508378,0.699006020085879));
#9570=CARTESIAN_POINT('Ctrl Pts',(4.50000126278178,1.30915682219698,0.697118891599074));
#9571=CARTESIAN_POINT('Ctrl Pts',(4.50000159346398,1.31346013814185,0.696056467716811));
#9572=CARTESIAN_POINT('Ctrl Pts',(4.50000189442328,1.31769890045703,0.694709922559592));
#9573=CARTESIAN_POINT('Ctrl Pts',(4.50000208642664,1.32184639782974,0.693090275295953));
#9574=CARTESIAN_POINT('Ctrl Pts',(4.50000243009859,1.32927011415192,0.690191225399894));
#9575=CARTESIAN_POINT('Ctrl Pts',(4.50000235826664,1.33632110693134,0.686451804482762));
#9576=CARTESIAN_POINT('Ctrl Pts',(4.50000192249634,1.34285330390028,0.681953677325188));
#9577=CARTESIAN_POINT('Ctrl Pts',(4.5000016824508,1.3464515866709,0.679475868782656));
#9578=CARTESIAN_POINT('Ctrl Pts',(4.50000134086274,1.34989218134371,0.676766953538005));
#9579=CARTESIAN_POINT('Ctrl Pts',(4.50000103767597,1.35314674504257,0.67383503027087));
#9580=CARTESIAN_POINT('Ctrl Pts',(4.50000074242034,1.35631617169348,0.670979804009792));
#9581=CARTESIAN_POINT('Ctrl Pts',(4.50000047986374,1.35928994516467,0.667930335702103));
#9582=CARTESIAN_POINT('Ctrl Pts',(4.5000004798165,1.36204555935344,0.66469809744354));
#9583=CARTESIAN_POINT('Ctrl Pts',(4.5000004797289,1.36715559606013,0.658704204607119));
#9584=CARTESIAN_POINT('Ctrl Pts',(4.50000128456446,1.3715183542993,0.652083197653858));
#9585=CARTESIAN_POINT('Ctrl Pts',(4.50000155892095,1.37507421485048,0.645000595057188));
#9586=CARTESIAN_POINT('Ctrl Pts',(4.50000158702893,1.37543851484667,0.644274978272754));
#9587=CARTESIAN_POINT('Ctrl Pts',(4.50000161091379,1.37579430519483,0.643544496675346));
#9588=CARTESIAN_POINT('Ctrl Pts',(4.50000163009343,1.37614149316233,0.642809317076966));
#9589=CARTESIAN_POINT('Ctrl Pts',(4.50000181728783,1.37953006709248,0.635633923185928));
#9590=CARTESIAN_POINT('Ctrl Pts',(4.50000140772507,1.38206400387968,0.628095594687559));
#9591=CARTESIAN_POINT('Ctrl Pts',(4.50000081194859,1.38368993781387,0.620362729373495));
#9592=CARTESIAN_POINT('Ctrl Pts',(4.50000042990035,1.38473258588096,0.615403944208116));
#9593=CARTESIAN_POINT('Ctrl Pts',(4.49999999988018,1.38540098970406,0.610364492806037));
#9594=CARTESIAN_POINT('Ctrl Pts',(4.50000000014037,1.38566996330298,0.605286533623957));
#9595=CARTESIAN_POINT('',(4.5,-1.28575421950842,0.7));
#9596=CARTESIAN_POINT('',(4.5,-0.742407407407408,0.7));
#9597=CARTESIAN_POINT('',(4.5,-1.38566996325095,0.605286533624017));
#9598=CARTESIAN_POINT('Ctrl Pts',(4.50000000014037,-1.38566996330298,0.605286533623957));
#9599=CARTESIAN_POINT('Ctrl Pts',(4.49999999973491,-1.38525081272033,0.613199687771457));
#9600=CARTESIAN_POINT('Ctrl Pts',(4.50000095642016,-1.38386419754969,0.62102180968747));
#9601=CARTESIAN_POINT('Ctrl Pts',(4.50000138305812,-1.38159414679432,0.628592503408469));
#9602=CARTESIAN_POINT('Ctrl Pts',(4.50000162118259,-1.38032713666619,0.632818023740444));
#9603=CARTESIAN_POINT('Ctrl Pts',(4.50000172745986,-1.37878391728058,0.636965253716347));
#9604=CARTESIAN_POINT('Ctrl Pts',(4.50000166716583,-1.37697237493585,0.641004309729874));
#9605=CARTESIAN_POINT('Ctrl Pts',(4.50000155916287,-1.37372741146613,0.648239354085419));
#9606=CARTESIAN_POINT('Ctrl Pts',(4.50000084040372,-1.36965973349804,0.655049237033139));
#9607=CARTESIAN_POINT('Ctrl Pts',(4.50000056390271,-1.36483316768901,0.661270759279915));
#9608=CARTESIAN_POINT('Ctrl Pts',(4.50000051219424,-1.36393055121024,0.662434246679675));
#9609=CARTESIAN_POINT('Ctrl Pts',(4.50000048023544,-1.3630012658104,0.663577087492372));
#9610=CARTESIAN_POINT('Ctrl Pts',(4.50000048056391,-1.36204555937839,0.664698097443534));
#9611=CARTESIAN_POINT('Ctrl Pts',(4.50000048121673,-1.36014610273268,0.666926093123284));
#9612=CARTESIAN_POINT('Ctrl Pts',(4.50000060829837,-1.35814231322364,0.669067903674665));
#9613=CARTESIAN_POINT('Ctrl Pts',(4.50000078085101,-1.35604151212276,0.671119765431539));
#9614=CARTESIAN_POINT('Ctrl Pts',(4.50000124774248,-1.3503571825734,0.676671675324794));
#9615=CARTESIAN_POINT('Ctrl Pts',(4.50000197143062,-1.34402953514766,0.681505303070731));
#9616=CARTESIAN_POINT('Ctrl Pts',(4.50000220836427,-1.33722229030693,0.685566265232058));
#9617=CARTESIAN_POINT('Ctrl Pts',(4.50000235894787,-1.33289593407788,0.688147216755564));
#9618=CARTESIAN_POINT('Ctrl Pts',(4.50000234488938,-1.32837489877041,0.690415387400166));
#9619=CARTESIAN_POINT('Ctrl Pts',(4.50000216490635,-1.32369554581057,0.69234752884452));
#9620=CARTESIAN_POINT('Ctrl Pts',(4.50000188343739,-1.31637767466938,0.695369135087455));
#9621=CARTESIAN_POINT('Ctrl Pts',(4.50000119588393,-1.3087575932273,0.697536490026807));
#9622=CARTESIAN_POINT('Ctrl Pts',(4.50000064127173,-1.30098224657147,0.698779892333419));
#9623=CARTESIAN_POINT('Ctrl Pts',(4.50000028296845,-1.29595903898196,0.699583183579437));
#9624=CARTESIAN_POINT('Ctrl Pts',(4.5,-1.29087043558603,0.7));
#9625=CARTESIAN_POINT('Ctrl Pts',(4.5,-1.28575421950843,0.7));
#9626=CARTESIAN_POINT('',(4.5,-1.41772989878425,0.));
#9627=CARTESIAN_POINT('Ctrl Pts',(4.5,-1.41772989878425,0.));
#9628=CARTESIAN_POINT('Ctrl Pts',(4.5,-1.41239649634988,0.100698149937961));
#9629=CARTESIAN_POINT('Ctrl Pts',(4.5,-1.40706297966336,0.201396293824709));
#9630=CARTESIAN_POINT('Ctrl Pts',(4.5,-1.39637633579674,0.403158471769294));
#9631=CARTESIAN_POINT('Ctrl Pts',(4.5,-1.39102320777973,0.504222505781934));
#9632=CARTESIAN_POINT('Ctrl Pts',(4.5,-1.38566996325095,0.605286533624017));
#9633=CARTESIAN_POINT('',(4.5,-1.48481481481482,0.));
#9634=CARTESIAN_POINT('Origin',(1.1,-1.39290118819044,0.));
#9635=CARTESIAN_POINT('',(1.1,1.324891758307,0.));
#9636=CARTESIAN_POINT('',(1.1,-1.39290118819044,0.));
#9637=CARTESIAN_POINT('',(1.10000000295569,1.29254692766489,0.605334652628491));
#9638=CARTESIAN_POINT('Ctrl Pts',(1.10000000295569,1.29254692766489,0.605334652628491));
#9639=CARTESIAN_POINT('Ctrl Pts',(1.10000000295569,1.29794978210809,0.504228164786351));
#9640=CARTESIAN_POINT('Ctrl Pts',(1.1,1.30335245345465,0.403121008362245));
#9641=CARTESIAN_POINT('Ctrl Pts',(1.1,1.31413403739463,0.20134322693425));
#9642=CARTESIAN_POINT('Ctrl Pts',(1.1,1.31951302132877,0.100671299071668));
#9643=CARTESIAN_POINT('Ctrl Pts',(1.1,1.324891758307,0.));
#9644=CARTESIAN_POINT('Ctrl Pts',(1.1,1.19266190204553,0.7));
#9645=CARTESIAN_POINT('Ctrl Pts',(1.1,1.20057109129252,0.7));
#9646=CARTESIAN_POINT('Ctrl Pts',(1.10000046829629,1.20841685974333,0.699006220526237));
#9647=CARTESIAN_POINT('Ctrl Pts',(1.10000087277688,1.21605887983377,0.697119382842322));
#9648=CARTESIAN_POINT('Ctrl Pts',(1.10000109992184,1.22035042410288,0.696059787689036));
#9649=CARTESIAN_POINT('Ctrl Pts',(1.10000130563842,1.22457776983048,0.694717521940989));
#9650=CARTESIAN_POINT('Ctrl Pts',(1.10000143498593,1.22871439246446,0.693103507978966));
#9651=CARTESIAN_POINT('Ctrl Pts',(1.10000166711622,1.23613807995602,0.690206957744321));
#9652=CARTESIAN_POINT('Ctrl Pts',(1.10000160692769,1.24318920265812,0.686469797174223));
#9653=CARTESIAN_POINT('Ctrl Pts',(1.10000129432656,1.24972159507123,0.681973692132557));
#9654=CARTESIAN_POINT('Ctrl Pts',(1.10000112259081,1.25331033895651,0.679503636989594));
#9655=CARTESIAN_POINT('Ctrl Pts',(1.10000088087184,1.25674225826706,0.676803638555143));
#9656=CARTESIAN_POINT('Ctrl Pts',(1.10000066684112,1.25998923415267,0.673881729486736));
#9657=CARTESIAN_POINT('Ctrl Pts',(1.100000457217,1.26316935916797,0.671019978599686));
#9658=CARTESIAN_POINT('Ctrl Pts',(1.1000002715704,1.26615273734033,0.667962699881477));
#9659=CARTESIAN_POINT('Ctrl Pts',(1.1000002731257,1.2689166530284,0.664721467295484));
#9660=CARTESIAN_POINT('Ctrl Pts',(1.10000027600127,1.2740268283512,0.658728785663437));
#9661=CARTESIAN_POINT('Ctrl Pts',(1.10000085014601,1.27838972527875,0.652108677049879));
#9662=CARTESIAN_POINT('Ctrl Pts',(1.1000010530947,1.28194599975408,0.64502688444408));
#9663=CARTESIAN_POINT('Ctrl Pts',(1.10000107362034,1.2823056710724,0.644310652415237));
#9664=CARTESIAN_POINT('Ctrl Pts',(1.10000109127028,1.28265705236355,0.643589678557342));
#9665=CARTESIAN_POINT('Ctrl Pts',(1.10000110571348,1.28300005475086,0.642864123553892));
#9666=CARTESIAN_POINT('Ctrl Pts',(1.10000124853573,1.28639184812822,0.635689442715943));
#9667=CARTESIAN_POINT('Ctrl Pts',(1.10000097361067,1.28892914698194,0.628151301589031));
#9668=CARTESIAN_POINT('Ctrl Pts',(1.10000056283738,1.29055881622654,0.620418355899457));
#9669=CARTESIAN_POINT('Ctrl Pts',(1.10000029930222,1.29160434466024,0.615457217544876));
#9670=CARTESIAN_POINT('Ctrl Pts',(1.0999999999818,1.29227543558766,0.610415225971447));
#9671=CARTESIAN_POINT('Ctrl Pts',(1.1000000000255,1.29254692753179,0.605334652628598));
#9672=CARTESIAN_POINT('',(1.10000000295569,-1.29254692766489,0.605334652628491));
#9673=CARTESIAN_POINT('Ctrl Pts',(1.1000000000255,-1.29254692753179,0.605334652628598));
#9674=CARTESIAN_POINT('Ctrl Pts',(1.09999999995744,-1.29212405100831,0.613248166229861));
#9675=CARTESIAN_POINT('Ctrl Pts',(1.10000066442022,-1.29073420569755,0.621070584654331));
#9676=CARTESIAN_POINT('Ctrl Pts',(1.10000095378343,-1.28846118610397,0.628641296001913));
#9677=CARTESIAN_POINT('Ctrl Pts',(1.10000111506646,-1.28719426797524,0.632861000698125));
#9678=CARTESIAN_POINT('Ctrl Pts',(1.10000118318417,-1.28565198202118,0.637002542581089));
#9679=CARTESIAN_POINT('Ctrl Pts',(1.10000113489265,-1.28384214455607,0.641036116698538));
#9680=CARTESIAN_POINT('Ctrl Pts',(1.10000104828677,-1.28059638744501,0.648269916488365));
#9681=CARTESIAN_POINT('Ctrl Pts',(1.10000053334783,-1.27652829029495,0.655078571385522));
#9682=CARTESIAN_POINT('Ctrl Pts',(1.10000033433257,-1.27170133822839,0.661298646557671));
#9683=CARTESIAN_POINT('Ctrl Pts',(1.10000029715544,-1.27079963749419,0.662460590217389));
#9684=CARTESIAN_POINT('Ctrl Pts',(1.10000027400485,-1.26987132743055,0.663601924550879));
#9685=CARTESIAN_POINT('Ctrl Pts',(1.10000027368829,-1.26891665304159,0.664721467295481));
#9686=CARTESIAN_POINT('Ctrl Pts',(1.10000027305905,-1.2670190620795,0.666946764442229));
#9687=CARTESIAN_POINT('Ctrl Pts',(1.10000036187052,-1.26501734165944,0.669086014589825));
#9688=CARTESIAN_POINT('Ctrl Pts',(1.10000048327469,-1.26291879257262,0.671135465892351));
#9689=CARTESIAN_POINT('Ctrl Pts',(1.10000081209565,-1.25723491092676,0.676686367091516));
#9690=CARTESIAN_POINT('Ctrl Pts',(1.10000132622062,-1.25090760500066,0.68151881845922));
#9691=CARTESIAN_POINT('Ctrl Pts',(1.10000150097561,-1.24410063152763,0.68557843671136));
#9692=CARTESIAN_POINT('Ctrl Pts',(1.10000161196703,-1.2397773464179,0.688156805381407));
#9693=CARTESIAN_POINT('Ctrl Pts',(1.1000016084534,-1.23525961544019,0.690422742497405));
#9694=CARTESIAN_POINT('Ctrl Pts',(1.10000148831111,-1.23058375131837,0.692353039195786));
#9695=CARTESIAN_POINT('Ctrl Pts',(1.10000130031927,-1.22326722442338,0.695373457954986));
#9696=CARTESIAN_POINT('Ctrl Pts',(1.1000008264887,-1.21564857658641,0.697539632783775));
#9697=CARTESIAN_POINT('Ctrl Pts',(1.10000044322439,-1.20787483729518,0.698781928831272));
#9698=CARTESIAN_POINT('Ctrl Pts',(1.1000001958084,-1.20285650563037,0.6995838921283));
#9699=CARTESIAN_POINT('Ctrl Pts',(1.1,-1.19777295102175,0.7));
#9700=CARTESIAN_POINT('Ctrl Pts',(1.1,-1.19266190204553,0.7));
#9701=CARTESIAN_POINT('',(1.1,-1.324891758307,0.));
#9702=CARTESIAN_POINT('Ctrl Pts',(1.1,-1.324891758307,0.));
#9703=CARTESIAN_POINT('Ctrl Pts',(1.1,-1.3195129727271,0.10067220872632));
#9704=CARTESIAN_POINT('Ctrl Pts',(1.1,-1.31413394019217,0.201345046154956));
#9705=CARTESIAN_POINT('Ctrl Pts',(1.1,-1.30335235623932,0.40312282767794));
#9706=CARTESIAN_POINT('Ctrl Pts',(1.10000000295569,-1.29794973349953,0.504229074424201));
#9707=CARTESIAN_POINT('Ctrl Pts',(1.10000000295569,-1.29254692766489,0.605334652628491));
#9708=CARTESIAN_POINT('',(1.1,-1.39290118819044,0.));
#9709=CARTESIAN_POINT('Origin',(0.199725906950915,-1.5,-0.0104671912485888));
#9710=CARTESIAN_POINT('',(0.200274469199584,1.20659878095028,0.));
#9711=CARTESIAN_POINT('',(0.200274469199585,-0.75,0.));
#9712=CARTESIAN_POINT('',(0.231993417893744,1.17491202960101,0.605233595624295));
#9713=CARTESIAN_POINT('Ctrl Pts',(0.200274469199584,1.20659878095028,-9.43255890062389E-18));
#9714=CARTESIAN_POINT('Ctrl Pts',(0.210847451958254,1.19603647956141,0.20174452921517));
#9715=CARTESIAN_POINT('Ctrl Pts',(0.221420434855641,1.18547422886796,0.403489061077219));
#9716=CARTESIAN_POINT('Ctrl Pts',(0.231993417893744,1.17491202960101,0.605233595624295));
#9717=CARTESIAN_POINT('',(0.231993417893744,-1.17491202960101,0.605233595624295));
#9718=CARTESIAN_POINT('',(0.231993417893744,-0.75,0.605233595624295));
#9719=CARTESIAN_POINT('',(0.200274469199584,-1.20659878095028,1.38777878078145E-17));
#9720=CARTESIAN_POINT('Ctrl Pts',(0.231993417893744,-1.17491202960101,0.605233595624295));
#9721=CARTESIAN_POINT('Ctrl Pts',(0.221420434855641,-1.18547422886796,0.40348906107722));
#9722=CARTESIAN_POINT('Ctrl Pts',(0.210847451958254,-1.19603647956141,0.20174452921517));
#9723=CARTESIAN_POINT('Ctrl Pts',(0.200274469199584,-1.20659878095028,2.0491421059976E-17));
#9724=CARTESIAN_POINT('',(0.200274469199585,-0.75,0.));
#9725=CARTESIAN_POINT('Origin',(6.87299528185878,-3.57834294608796E-18,
0.));
#9726=CARTESIAN_POINT('Ctrl Pts',(8.90000000000001,-1.62420669932031,-3.75133951679985E-17));
#9727=CARTESIAN_POINT('Ctrl Pts',(10.0682843079684,-1.69891080436391,-1.31961514553165E-7));
#9728=CARTESIAN_POINT('Ctrl Pts',(11.2345361392062,-1.79243531443695,-6.44452192334729E-8));
#9729=CARTESIAN_POINT('Ctrl Pts',(12.4000000002382,-1.91212902541327,2.95121624705651E-11));
#9730=CARTESIAN_POINT('Ctrl Pts',(12.4000000002382,1.91212902541327,2.95118849063386E-11));
#9731=CARTESIAN_POINT('Ctrl Pts',(11.2345361911441,1.79243531977099,-6.4445136166539E-8));
#9732=CARTESIAN_POINT('Ctrl Pts',(10.0682843567552,1.69891080748336,-1.31958638870612E-7));
#9733=CARTESIAN_POINT('Ctrl Pts',(8.9,1.62420669932031,6.39679281766448E-17));
#9734=CARTESIAN_POINT('',(8.7,1.61160179736194,0.));
#9735=CARTESIAN_POINT('',(8.7,1.68851851851852,0.));
#9736=CARTESIAN_POINT('Ctrl Pts',(8.70000000002062,1.61160179731554,-3.21507306454832E-13));
#9737=CARTESIAN_POINT('Ctrl Pts',(7.99734938728961,1.56795839277283,5.29471456843263E-9));
#9738=CARTESIAN_POINT('Ctrl Pts',(7.29393815910572,1.53097060499506,-6.44604909847991E-9));
#9739=CARTESIAN_POINT('Ctrl Pts',(6.58949465297818,1.49904250536939,-7.60372244394637E-9));
#9740=CARTESIAN_POINT('Ctrl Pts',(5.94302350041144,1.46974193664425,-8.66612477447903E-9));
#9741=CARTESIAN_POINT('Ctrl Pts',(5.29757001768168,1.44478244743454,1.79883147367388E-8));
#9742=CARTESIAN_POINT('Ctrl Pts',(4.65216233480351,1.42284617839366,3.84107779578714E-9));
#9743=CARTESIAN_POINT('Ctrl Pts',(4.60144142975536,1.4211222642714,2.72928337404163E-9));
#9744=CARTESIAN_POINT('Ctrl Pts',(4.55072080855761,1.41941704699729,1.44770501019496E-9));
#9745=CARTESIAN_POINT('Ctrl Pts',(4.50000000001737,1.41772989873549,-1.00876616052154E-12));
#9746=CARTESIAN_POINT('',(4.3,1.41116952203211,0.));
#9747=CARTESIAN_POINT('',(4.3,1.48481481481482,0.));
#9748=CARTESIAN_POINT('Ctrl Pts',(4.3,1.41116952203211,-1.0790522121662E-15));
#9749=CARTESIAN_POINT('Ctrl Pts',(3.23514221724601,1.37672428690534,3.20725535317031E-8));
#9750=CARTESIAN_POINT('Ctrl Pts',(2.16992716239601,1.34987955958158,4.63097810372671E-9));
#9751=CARTESIAN_POINT('Ctrl Pts',(1.10000000020726,1.32489175811528,-9.82792569252214E-12));
#9752=CARTESIAN_POINT('',(0.9,1.32024227787037,0.));
#9753=CARTESIAN_POINT('',(0.9,1.39290118819044,0.));
#9754=CARTESIAN_POINT('',(0.297857995688647,1.306435779838,0.));
#9755=CARTESIAN_POINT('Ctrl Pts',(0.9,1.32024227787037,-6.93889390390723E-18));
#9756=CARTESIAN_POINT('Ctrl Pts',(0.699470323836888,1.31560060380002,-4.72996299588896E-10));
#9757=CARTESIAN_POINT('Ctrl Pts',(0.498765843889866,1.3110112408976,-1.02277582142263E-13));
#9758=CARTESIAN_POINT('Ctrl Pts',(0.297857995688647,1.306435779838,-1.00157829096748E-16));
#9759=CARTESIAN_POINT('Ctrl Pts',(0.297857995688647,1.306435779838,-1.95156391047391E-17));
#9760=CARTESIAN_POINT('Ctrl Pts',(0.289922476296638,1.30625505685688,-1.46278605970555E-13));
#9761=CARTESIAN_POINT('Ctrl Pts',(0.282050301799808,1.30510306275878,-1.25203502999379E-6));
#9762=CARTESIAN_POINT('Ctrl Pts',(0.274405144964298,1.30305953674341,-1.39678564665046E-6));
#9763=CARTESIAN_POINT('Ctrl Pts',(0.269498922713003,1.30174811919849,-1.48967827287246E-6));
#9764=CARTESIAN_POINT('Ctrl Pts',(0.26468600784495,1.30006837070384,-1.17796618578504E-6));
#9765=CARTESIAN_POINT('Ctrl Pts',(0.260012701218123,1.29803054880949,-5.63923085528507E-7));
#9766=CARTESIAN_POINT('Ctrl Pts',(0.252740988282594,1.29485967708789,3.91534262267771E-7));
#9767=CARTESIAN_POINT('Ctrl Pts',(0.245891302634708,1.2908611961912,2.26944434681222E-6));
#9768=CARTESIAN_POINT('Ctrl Pts',(0.239629152465829,1.28609427281,1.73040332626933E-6));
#9769=CARTESIAN_POINT('Ctrl Pts',(0.238677421334952,1.28536978852616,1.6484790500646E-6));
#9770=CARTESIAN_POINT('Ctrl Pts',(0.23773930716971,1.28462746803483,1.50379952206709E-6));
#9771=CARTESIAN_POINT('Ctrl Pts',(0.236815449960777,1.28386742955246,1.27686598471174E-6));
#9772=CARTESIAN_POINT('Ctrl Pts',(0.233849259515119,1.28142720517261,5.48259784756267E-7));
#9773=CARTESIAN_POINT('Ctrl Pts',(0.231029859162728,1.27880446664625,-1.01231737317126E-6));
#9774=CARTESIAN_POINT('Ctrl Pts',(0.228365947504865,1.27601569667724,-2.73789903475208E-6));
#9775=CARTESIAN_POINT('Ctrl Pts',(0.222875659368053,1.2702680771449,-6.2943009513513E-6));
#9776=CARTESIAN_POINT('Ctrl Pts',(0.218108003769119,1.26388547870891,-1.02458913084139E-5));
#9777=CARTESIAN_POINT('Ctrl Pts',(0.214119068651703,1.25703104885628,-1.16727273233865E-5));
#9778=CARTESIAN_POINT('Ctrl Pts',(0.211608035823831,1.25271618840614,-1.25709199407453E-5));
#9779=CARTESIAN_POINT('Ctrl Pts',(0.209406266788438,1.24821342134138,-1.25531979180244E-5));
#9780=CARTESIAN_POINT('Ctrl Pts',(0.207536767894457,1.24355803714115,-1.16467700682383E-5));
#9781=CARTESIAN_POINT('Ctrl Pts',(0.204585779527196,1.23620955211972,-1.02159812889057E-5));
#9782=CARTESIAN_POINT('Ctrl Pts',(0.20249437279756,1.22856635796309,-6.44823334219156E-6));
#9783=CARTESIAN_POINT('Ctrl Pts',(0.201333199355162,1.22077498745768,-3.37414558979738E-6));
#9784=CARTESIAN_POINT('Ctrl Pts',(0.200635497716839,1.21609347152911,-1.5270519663277E-6));
#9785=CARTESIAN_POINT('Ctrl Pts',(0.200274469246579,1.21135795995708,-3.76748562593766E-12));
#9786=CARTESIAN_POINT('Ctrl Pts',(0.200274469199584,1.20659878095028,6.07153216591882E-18));
#9787=CARTESIAN_POINT('',(-2.81723893694256E-19,1.20714678905882,-2.77862675945125E-17));
#9788=CARTESIAN_POINT('',(0.,-1.5,0.));
#9789=CARTESIAN_POINT('',(0.292751161823634,1.50665779898694,0.));
#9790=CARTESIAN_POINT('Ctrl Pts',(0.292751161823634,1.50665779898694,-4.77048955893622E-17));
#9791=CARTESIAN_POINT('Ctrl Pts',(0.274916014309114,1.50625165707847,3.84528327419955E-12));
#9792=CARTESIAN_POINT('Ctrl Pts',(0.257184594685611,1.50420857033458,-2.03607170333744E-6));
#9793=CARTESIAN_POINT('Ctrl Pts',(0.239764500086274,1.50063675387888,-2.79213621391921E-6));
#9794=CARTESIAN_POINT('Ctrl Pts',(0.222116086584643,1.49701812291205,-3.55811018958082E-6));
#9795=CARTESIAN_POINT('Ctrl Pts',(0.204785660682177,1.49183000356027,-2.9511242418033E-6));
#9796=CARTESIAN_POINT('Ctrl Pts',(0.187998620502071,1.4851341555102,-6.80337370794577E-7));
#9797=CARTESIAN_POINT('Ctrl Pts',(0.185044527596802,1.48395585623842,-2.80736529130144E-7));
#9798=CARTESIAN_POINT('Ctrl Pts',(0.182107319868513,1.48273075079643,1.61255976403501E-7));
#9799=CARTESIAN_POINT('Ctrl Pts',(0.17918831289364,1.48145903083089,6.35063889779883E-7));
#9800=CARTESIAN_POINT('Ctrl Pts',(0.162608037952008,1.47423552404966,3.32634402063389E-6));
#9801=CARTESIAN_POINT('Ctrl Pts',(0.146760254055949,1.46557586252388,7.36741945499403E-6));
#9802=CARTESIAN_POINT('Ctrl Pts',(0.131860714325404,1.4555643673366,8.80872142158042E-6));
#9803=CARTESIAN_POINT('Ctrl Pts',(0.12416804976458,1.45039541073654,9.55286874158632E-6));
#9804=CARTESIAN_POINT('Ctrl Pts',(0.116728404005452,1.44486529627202,9.54902993357918E-6));
#9805=CARTESIAN_POINT('Ctrl Pts',(0.109574210210226,1.43898090192647,7.86258910610491E-6));
#9806=CARTESIAN_POINT('Ctrl Pts',(0.100675189791982,1.43166137062374,5.76484451217541E-6));
#9807=CARTESIAN_POINT('Ctrl Pts',(0.0922175942578585,1.42379373777092,1.07962821494929E-6));
#9808=CARTESIAN_POINT('Ctrl Pts',(0.0842272493232774,1.41542759110015,-4.17082519724513E-6));
#9809=CARTESIAN_POINT('Ctrl Pts',(0.0719003514327883,1.40252093480537,-1.22708263387205E-5));
#9810=CARTESIAN_POINT('Ctrl Pts',(0.0607923942774574,1.38854365509349,-2.1446290640466E-5));
#9811=CARTESIAN_POINT('Ctrl Pts',(0.0509667079859164,1.37370740939602,-2.73088451608079E-5));
#9812=CARTESIAN_POINT('Ctrl Pts',(0.040988527714452,1.35864090617899,-3.32623861267576E-5));
#9813=CARTESIAN_POINT('Ctrl Pts',(0.0323319291028794,1.34268723517955,-3.58272570146011E-5));
#9814=CARTESIAN_POINT('Ctrl Pts',(0.0251054147216294,1.32603775378173,-3.42048160832586E-5));
#9815=CARTESIAN_POINT('Ctrl Pts',(0.0239557673766072,1.32338903116455,-3.39467061825833E-5));
#9816=CARTESIAN_POINT('Ctrl Pts',(0.022842414085455,1.32072266145131,-3.35898145907185E-5));
#9817=CARTESIAN_POINT('Ctrl Pts',(0.0217659098422027,1.31803938112476,-3.31388957009043E-5));
#9818=CARTESIAN_POINT('Ctrl Pts',(0.0146851456525434,1.30038996137917,-3.01729526055095E-5));
#9819=CARTESIAN_POINT('Ctrl Pts',(0.00925910545076598,1.282173175788,-2.28911926108039E-5));
#9820=CARTESIAN_POINT('Ctrl Pts',(0.0055880418397064,1.26361786690427,-1.53360241296986E-5));
#9821=CARTESIAN_POINT('Ctrl Pts',(0.00217213684284492,1.24635225152695,
-8.30598038733772E-6));
#9822=CARTESIAN_POINT('Ctrl Pts',(0.000275638047107462,1.2287919996398,
-1.11502351997496E-6));
#9823=CARTESIAN_POINT('Ctrl Pts',(2.78020181985954E-5,1.21111091902543,
-1.13803743790751E-7));
#9824=CARTESIAN_POINT('Ctrl Pts',(9.289355304618E-6,1.20979019141994,-3.90154078055202E-8));
#9825=CARTESIAN_POINT('Ctrl Pts',(3.5054796412911E-11,1.20846879032832,
-2.82152417201308E-12));
#9826=CARTESIAN_POINT('Ctrl Pts',(6.5594231435373E-18,1.20714678905882,
2.42861286636753E-17));
#9827=CARTESIAN_POINT('',(12.8678148030684,2.16300527278356,0.));
#9828=CARTESIAN_POINT('Ctrl Pts',(0.292751161823634,1.50665779898694,0.));
#9829=CARTESIAN_POINT('Ctrl Pts',(4.48443904223854,1.60211086545473,0.));
#9830=CARTESIAN_POINT('Ctrl Pts',(8.67612692265345,1.70561506876628,0.));
#9831=CARTESIAN_POINT('Ctrl Pts',(12.8678148030684,2.16300527278356,0.));
#9832=CARTESIAN_POINT('',(13.2,1.86519007666192,1.29914761427265E-16));
#9833=CARTESIAN_POINT('Ctrl Pts',(13.2,1.86519007666192,1.40512601554121E-16));
#9834=CARTESIAN_POINT('Ctrl Pts',(13.2000000013352,1.88296731840607,9.35191444695304E-11));
#9835=CARTESIAN_POINT('Ctrl Pts',(13.1983511006715,1.90064589040826,-4.81925060583158E-6));
#9836=CARTESIAN_POINT('Ctrl Pts',(13.1951709302004,1.91804121845656,-9.22684518112407E-6));
#9837=CARTESIAN_POINT('Ctrl Pts',(13.1919252271695,1.93579500539423,-1.37252653764835E-5));
#9838=CARTESIAN_POINT('Ctrl Pts',(13.1870840836913,1.95325521073227,-1.77396479500911E-5));
#9839=CARTESIAN_POINT('Ctrl Pts',(13.1807207319279,1.9702167899609,-1.88895599539727E-5));
#9840=CARTESIAN_POINT('Ctrl Pts',(13.179605107926,1.97319049715201,-1.90911627380646E-5));
#9841=CARTESIAN_POINT('Ctrl Pts',(13.1784425783122,1.97614882406338,-1.92137058190342E-5));
#9842=CARTESIAN_POINT('Ctrl Pts',(13.1772333926356,1.97909058504493,-1.92562174744009E-5));
#9843=CARTESIAN_POINT('Ctrl Pts',(13.1703491364924,1.99583891121373,-1.94982490583826E-5));
#9844=CARTESIAN_POINT('Ctrl Pts',(13.1620175712498,2.0119031422279,-1.67925698753361E-5));
#9845=CARTESIAN_POINT('Ctrl Pts',(13.1523342210936,2.02708796667103,-1.30402710852334E-5));
#9846=CARTESIAN_POINT('Ctrl Pts',(13.1443502942575,2.03960786168842,-9.94649893779315E-6));
#9847=CARTESIAN_POINT('Ctrl Pts',(13.1354462980072,2.05153020544825,-6.18593217696112E-6));
#9848=CARTESIAN_POINT('Ctrl Pts',(13.1256528604983,2.06273196126272,-4.73977425690188E-6));
#9849=CARTESIAN_POINT('Ctrl Pts',(13.1217453950533,2.06720132901318,-4.16277439392992E-6));
#9850=CARTESIAN_POINT('Ctrl Pts',(13.1176961215346,2.07155579183536,-3.97575052791371E-6));
#9851=CARTESIAN_POINT('Ctrl Pts',(13.1135113749213,2.07579033931164,-3.99023031318383E-6));
#9852=CARTESIAN_POINT('Ctrl Pts',(13.1009362730034,2.08851509208914,-4.03374185458576E-6));
#9853=CARTESIAN_POINT('Ctrl Pts',(13.0872516297578,2.10004749226926,-5.60236028337187E-6));
#9854=CARTESIAN_POINT('Ctrl Pts',(13.0726646436523,2.11028882659185,-6.03124820804926E-6));
#9855=CARTESIAN_POINT('Ctrl Pts',(13.0580194031224,2.12057106059247,-6.46184893473862E-6));
#9856=CARTESIAN_POINT('Ctrl Pts',(13.0424632957183,2.12955278528135,-5.76500392338198E-6));
#9857=CARTESIAN_POINT('Ctrl Pts',(13.0261754841647,2.13709349482706,-4.98347139369932E-6));
#9858=CARTESIAN_POINT('Ctrl Pts',(13.0233759049672,2.13838960594114,-4.84914013593099E-6));
#9859=CARTESIAN_POINT('Ctrl Pts',(13.0205546633935,2.13964302898522,-4.72077764982159E-6));
#9860=CARTESIAN_POINT('Ctrl Pts',(13.0177126224567,2.14085289970554,-4.61407510358037E-6));
#9861=CARTESIAN_POINT('Ctrl Pts',(13.0148367726024,2.14207716304734,-4.50610322390289E-6));
#9862=CARTESIAN_POINT('Ctrl Pts',(13.0119432782921,2.14325527660784,-4.42172619954107E-6));
#9863=CARTESIAN_POINT('Ctrl Pts',(13.0090331608036,2.14438664763146,-4.38057543634576E-6));
#9864=CARTESIAN_POINT('Ctrl Pts',(12.9922536897216,2.1509100294015,-4.14330390220891E-6));
#9865=CARTESIAN_POINT('Ctrl Pts',(12.9749229882599,2.15588345271621,-5.05640020348117E-6));
#9866=CARTESIAN_POINT('Ctrl Pts',(12.9572550825995,2.15928949382789,-4.85686529648217E-6));
#9867=CARTESIAN_POINT('Ctrl Pts',(12.9529252316797,2.16012420794307,-4.80796553341985E-6));
#9868=CARTESIAN_POINT('Ctrl Pts',(12.9485750628159,2.16086455090717,-4.70814629363608E-6));
#9869=CARTESIAN_POINT('Ctrl Pts',(12.944207640703,2.16150979950679,-4.55317442353944E-6));
#9870=CARTESIAN_POINT('Ctrl Pts',(12.9263774359968,2.16414405704371,-3.92049452767182E-6));
#9871=CARTESIAN_POINT('Ctrl Pts',(12.9083632163621,2.16518216214944,-2.15504024707585E-6));
#9872=CARTESIAN_POINT('Ctrl Pts',(12.8903762705535,2.16459816844574,-9.12104093693782E-7));
#9873=CARTESIAN_POINT('Ctrl Pts',(12.8828459063217,2.16435367528137,-3.91739933400607E-7));
#9874=CARTESIAN_POINT('Ctrl Pts',(12.8753202361859,2.1638242536466,5.87463683432524E-12));
#9875=CARTESIAN_POINT('Ctrl Pts',(12.8678148030684,2.16300527278357,2.8796409701215E-16));
#9876=CARTESIAN_POINT('',(13.2,-1.86519007666192,1.11326398357188E-16));
#9877=CARTESIAN_POINT('',(13.2,2.2,0.));
#9878=CARTESIAN_POINT('',(12.8678148030684,-2.16300527278356,1.38777878078145E-17));
#9879=CARTESIAN_POINT('Ctrl Pts',(12.8678148030684,-2.16300527278357,2.56739074444567E-16));
#9880=CARTESIAN_POINT('Ctrl Pts',(12.8854929372559,-2.16493428409685,8.24591542686399E-11));
#9881=CARTESIAN_POINT('Ctrl Pts',(12.9032520674897,-2.16521372082443,-4.52295339524789E-6));
#9882=CARTESIAN_POINT('Ctrl Pts',(12.9208958607904,-2.1639404182545,-8.68231213275745E-6));
#9883=CARTESIAN_POINT('Ctrl Pts',(12.9389012534027,-2.16264102008682,-1.29269145154966E-5));
#9884=CARTESIAN_POINT('Ctrl Pts',(12.9567880250381,-2.15972433317902,-1.67278855193166E-5));
#9885=CARTESIAN_POINT('Ctrl Pts',(12.9743443410528,-2.15524079327399,-1.78237954457702E-5));
#9886=CARTESIAN_POINT('Ctrl Pts',(12.9774431846623,-2.15444940919484,-1.80172331504298E-5));
#9887=CARTESIAN_POINT('Ctrl Pts',(12.9805316913262,-2.15360908525727,-1.81351031595367E-5));
#9888=CARTESIAN_POINT('Ctrl Pts',(12.9836086301392,-2.15271994254544,-1.81766625580856E-5));
#9889=CARTESIAN_POINT('Ctrl Pts',(13.0010041030966,-2.14769317440371,-1.84116186093898E-5));
#9890=CARTESIAN_POINT('Ctrl Pts',(13.017876958431,-2.14115457229109,-1.5854618169158E-5));
#9891=CARTESIAN_POINT('Ctrl Pts',(13.0340226638693,-2.13317744288338,-1.23136839993165E-5));
#9892=CARTESIAN_POINT('Ctrl Pts',(13.0473215411186,-2.12660684953271,-9.39709115965876E-6));
#9893=CARTESIAN_POINT('Ctrl Pts',(13.060127470267,-2.11905920305061,-5.85016632862467E-6));
#9894=CARTESIAN_POINT('Ctrl Pts',(13.0723151314263,-2.11055132433008,-4.53327195050794E-6));
#9895=CARTESIAN_POINT('Ctrl Pts',(13.0772147086919,-2.10713106111368,-4.00386555564548E-6));
#9896=CARTESIAN_POINT('Ctrl Pts',(13.0820141951123,-2.10355537352593,-3.85636210984559E-6));
#9897=CARTESIAN_POINT('Ctrl Pts',(13.0867078006727,-2.0998301147952,-3.90248451975241E-6));
#9898=CARTESIAN_POINT('Ctrl Pts',(13.1007249787291,-2.08870484782034,-4.04022639510273E-6));
#9899=CARTESIAN_POINT('Ctrl Pts',(13.1136765748478,-2.07634683247102,-5.5945154994439E-6));
#9900=CARTESIAN_POINT('Ctrl Pts',(13.1254414850725,-2.06295113861397,-5.97495381195624E-6));
#9901=CARTESIAN_POINT('Ctrl Pts',(13.1372476314214,-2.04950849272046,-6.35672556443159E-6));
#9902=CARTESIAN_POINT('Ctrl Pts',(13.1478597809499,-2.03501968083851,-5.56609061204695E-6));
#9903=CARTESIAN_POINT('Ctrl Pts',(13.1571184147632,-2.01964723728874,-4.75455255839871E-6));
#9904=CARTESIAN_POINT('Ctrl Pts',(13.158708901902,-2.01700649414547,-4.61514313115074E-6));
#9905=CARTESIAN_POINT('Ctrl Pts',(13.1602593369672,-2.01433961799121,-4.48389992381974E-6));
#9906=CARTESIAN_POINT('Ctrl Pts',(13.1617687665475,-2.01164737048868,-4.37752847101542E-6));
#9907=CARTESIAN_POINT('Ctrl Pts',(13.1632768494098,-2.00895752501823,-4.27125192317111E-6));
#9908=CARTESIAN_POINT('Ctrl Pts',(13.164742106841,-2.00624572954308,-4.19089851494128E-6));
#9909=CARTESIAN_POINT('Ctrl Pts',(13.1661638648313,-2.00351289682408,-4.15637526360595E-6));
#9910=CARTESIAN_POINT('Ctrl Pts',(13.1744716670281,-1.98754405133797,-3.95464448717833E-6));
#9911=CARTESIAN_POINT('Ctrl Pts',(13.181298057795,-1.97085874357403,-5.01850453361653E-6));
#9912=CARTESIAN_POINT('Ctrl Pts',(13.1866022393826,-1.95366776591112,-4.89891140766866E-6));
#9913=CARTESIAN_POINT('Ctrl Pts',(13.1879075264936,-1.94943729958961,-4.86948116225E-6));
#9914=CARTESIAN_POINT('Ctrl Pts',(13.1891204013114,-1.94517611908519,-4.78523710928743E-6));
#9915=CARTESIAN_POINT('Ctrl Pts',(13.1902397948733,-1.94088722910442,-4.64104147683466E-6));
#9916=CARTESIAN_POINT('Ctrl Pts',(13.1947901580114,-1.92345278286841,-4.05488258426869E-6));
#9917=CARTESIAN_POINT('Ctrl Pts',(13.1977733658442,-1.90566244769967,-2.24449026644408E-6));
#9918=CARTESIAN_POINT('Ctrl Pts',(13.1991406030032,-1.88772335428786,-9.50757284845071E-7));
#9919=CARTESIAN_POINT('Ctrl Pts',(13.1997114533543,-1.8802334044254,-4.10596478211383E-7));
#9920=CARTESIAN_POINT('Ctrl Pts',(13.2000000000958,-1.87271737110067,6.9401096738129E-12));
#9921=CARTESIAN_POINT('Ctrl Pts',(13.2,-1.86519007666192,1.81278603239576E-16));
#9922=CARTESIAN_POINT('',(0.292751161823634,-1.50665779898694,-1.38777878078145E-17));
#9923=CARTESIAN_POINT('Ctrl Pts',(12.8678148030684,-2.16300527278356,0.));
#9924=CARTESIAN_POINT('Ctrl Pts',(8.67612692265345,-1.70561506876628,0.));
#9925=CARTESIAN_POINT('Ctrl Pts',(4.48443904223854,-1.60211086545473,0.));
#9926=CARTESIAN_POINT('Ctrl Pts',(0.292751161823634,-1.50665779898694,0.));
#9927=CARTESIAN_POINT('',(4.02814324098787E-18,-1.20714678905882,5.54818711994559E-17));
#9928=CARTESIAN_POINT('Ctrl Pts',(-2.22044604925031E-16,-1.20714678905882,
-3.98986399474666E-17));
#9929=CARTESIAN_POINT('Ctrl Pts',(2.12382277713531E-10,-1.2249878157372,
-1.35440422383976E-12));
#9930=CARTESIAN_POINT('Ctrl Pts',(0.00163882612763064,-1.24276245549475,
-1.96699749426327E-6));
#9931=CARTESIAN_POINT('Ctrl Pts',(0.00481304415265273,-1.26026068126938,
-2.66007142975038E-6));
#9932=CARTESIAN_POINT('Ctrl Pts',(0.00802873944670128,-1.27798755504872,
-3.36220171040687E-6));
#9933=CARTESIAN_POINT('Ctrl Pts',(0.0128206026099745,-1.29543230475431,
-2.69550948014298E-6));
#9934=CARTESIAN_POINT('Ctrl Pts',(0.0191320595672371,-1.31236817798419,
-4.00401478067381E-7));
#9935=CARTESIAN_POINT('Ctrl Pts',(0.0202443702650641,-1.31535290133701,
4.0809101773195E-9));
#9936=CARTESIAN_POINT('Ctrl Pts',(0.0214039964883031,-1.3183217636574,4.5005107558061E-7));
#9937=CARTESIAN_POINT('Ctrl Pts',(0.0226107760969305,-1.32127343934773,
9.26779280916758E-7));
#9938=CARTESIAN_POINT('Ctrl Pts',(0.0294548697216842,-1.33801348419941,
3.63048130534217E-6));
#9939=CARTESIAN_POINT('Ctrl Pts',(0.0377511831708778,-1.35405403406083,
7.64722139837078E-6));
#9940=CARTESIAN_POINT('Ctrl Pts',(0.0474204318104353,-1.36917746582299,
9.03443059383348E-6));
#9941=CARTESIAN_POINT('Ctrl Pts',(0.0524109755304394,-1.37698305136733,
9.75040433665629E-6));
#9942=CARTESIAN_POINT('Ctrl Pts',(0.0577680562174045,-1.38454410063597,
9.71159147480002E-6));
#9943=CARTESIAN_POINT('Ctrl Pts',(0.0634855547170043,-1.39182806229354,
7.98761394269614E-6));
#9944=CARTESIAN_POINT('Ctrl Pts',(0.0706048733905122,-1.40089791062835,
5.84095042579577E-6));
#9945=CARTESIAN_POINT('Ctrl Pts',(0.0782829434694699,-1.40953838460506,
1.09773645972912E-6));
#9946=CARTESIAN_POINT('Ctrl Pts',(0.0864706998703675,-1.41772246232928,
-4.21049985396393E-6));
#9947=CARTESIAN_POINT('Ctrl Pts',(0.0990944981487371,-1.43034058886193,
-1.2394683793612E-5));
#9948=CARTESIAN_POINT('Ctrl Pts',(0.112816484288725,-1.44176429483685,-2.16481703631134E-5));
#9949=CARTESIAN_POINT('Ctrl Pts',(0.127426518150943,-1.45192534842919,-2.7562374581111E-5));
#9950=CARTESIAN_POINT('Ctrl Pts',(0.142261949549145,-1.46224316253723,-3.35678206860622E-5));
#9951=CARTESIAN_POINT('Ctrl Pts',(0.158014355623482,-1.47125989363127,-3.6155642403295E-5));
#9952=CARTESIAN_POINT('Ctrl Pts',(0.17449494651519,-1.47886261331763,-3.45187637154371E-5));
#9953=CARTESIAN_POINT('Ctrl Pts',(0.177115379630184,-1.48007145458801,-3.42584981007467E-5));
#9954=CARTESIAN_POINT('Ctrl Pts',(0.179754261386328,-1.48124444832217,-3.38986806574493E-5));
#9955=CARTESIAN_POINT('Ctrl Pts',(0.18241086941249,-1.48238102342202,-3.34441145409493E-5));
#9956=CARTESIAN_POINT('Ctrl Pts',(0.199890279181845,-1.48985922935543,-3.04532527580594E-5));
#9957=CARTESIAN_POINT('Ctrl Pts',(0.217974246898519,-1.49569663469242,-2.31073027206853E-5));
#9958=CARTESIAN_POINT('Ctrl Pts',(0.236436446036386,-1.49978781870256,-1.54828395726751E-5));
#9959=CARTESIAN_POINT('Ctrl Pts',(0.253618559172887,-1.50359533838099,-8.38702246898572E-6));
#9960=CARTESIAN_POINT('Ctrl Pts',(0.271129804961754,-1.50589051664322,-1.1237837803371E-6));
#9961=CARTESIAN_POINT('Ctrl Pts',(0.288799387895208,-1.50654014509364,-1.14426782679271E-7));
#9962=CARTESIAN_POINT('Ctrl Pts',(0.290115790923368,-1.5065885431154,-3.92285953074499E-8));
#9963=CARTESIAN_POINT('Ctrl Pts',(0.291433072638222,-1.50662778343727,-2.32210426557352E-12));
#9964=CARTESIAN_POINT('Ctrl Pts',(0.292751161823634,-1.50665779898694,2.86229373536173E-17));
#9965=CARTESIAN_POINT('',(0.,-1.5,0.));
#9966=CARTESIAN_POINT('',(0.297857995688647,-1.306435779838,0.));
#9967=CARTESIAN_POINT('Ctrl Pts',(0.200274469199585,-1.20659878095028,-5.63785129692462E-18));
#9968=CARTESIAN_POINT('Ctrl Pts',(0.200274469233139,-1.21453676310593,-8.71436967499621E-13));
#9969=CARTESIAN_POINT('Ctrl Pts',(0.201246859971722,-1.22243356087926,-1.21395871814677E-6));
#9970=CARTESIAN_POINT('Ctrl Pts',(0.203115675186186,-1.23012372049816,-1.3343733317444E-6));
#9971=CARTESIAN_POINT('Ctrl Pts',(0.204315340901654,-1.23506033529553,-1.41167219064517E-6));
#9972=CARTESIAN_POINT('Ctrl Pts',(0.20588557457721,-1.23991201018842,-1.08820351238587E-6));
#9973=CARTESIAN_POINT('Ctrl Pts',(0.207817175189242,-1.24463217458037,-4.7123943162984E-7));
#9974=CARTESIAN_POINT('Ctrl Pts',(0.210821635148072,-1.25197403646754,4.8840194822981E-7));
#9975=CARTESIAN_POINT('Ctrl Pts',(0.214662962735955,-1.25891288736431,2.34840446672759E-6));
#9976=CARTESIAN_POINT('Ctrl Pts',(0.219285851586231,-1.26528190572196,1.77850405974346E-6));
#9977=CARTESIAN_POINT('Ctrl Pts',(0.219987799701267,-1.26624898941694,1.69196931287913E-6));
#9978=CARTESIAN_POINT('Ctrl Pts',(0.220707854727247,-1.26720289123473,1.54254180957111E-6));
#9979=CARTESIAN_POINT('Ctrl Pts',(0.221445913570039,-1.26814297034805,1.31084431541716E-6));
#9980=CARTESIAN_POINT('Ctrl Pts',(0.223819423285066,-1.27116615329633,5.65732650279818E-7));
#9981=CARTESIAN_POINT('Ctrl Pts',(0.226378993511503,-1.27404655624932,-1.0141799309673E-6));
#9982=CARTESIAN_POINT('Ctrl Pts',(0.229108317341547,-1.27677508245113,-2.75886047820546E-6));
#9983=CARTESIAN_POINT('Ctrl Pts',(0.234729699316268,-1.28239482161129,-6.35224711555937E-6));
#9984=CARTESIAN_POINT('Ctrl Pts',(0.241002345945823,-1.28730653457646,-1.03364935932408E-5));
#9985=CARTESIAN_POINT('Ctrl Pts',(0.247764463424355,-1.29145035967733,-1.17765252099068E-5));
#9986=CARTESIAN_POINT('Ctrl Pts',(0.25202072563572,-1.29405859685204,-1.26829206064147E-5));
#9987=CARTESIAN_POINT('Ctrl Pts',(0.25647185453211,-1.29636195369988,-1.26655904667795E-5));
#9988=CARTESIAN_POINT('Ctrl Pts',(0.261083107941716,-1.29833661269995,-1.17517412599227E-5));
#9989=CARTESIAN_POINT('Ctrl Pts',(0.268362152520619,-1.30145368947124,-1.0309194402435E-5));
#9990=CARTESIAN_POINT('Ctrl Pts',(0.275955349537693,-1.30371808689536,-6.50743389458559E-6));
#9991=CARTESIAN_POINT('Ctrl Pts',(0.283717840216357,-1.30505580179168,-3.40467605837577E-6));
#9992=CARTESIAN_POINT('Ctrl Pts',(0.288379557365255,-1.3058591584372,-1.54133347766382E-6));
#9993=CARTESIAN_POINT('Ctrl Pts',(0.293102847896135,-1.30632748638856,-3.09915230996644E-12));
#9994=CARTESIAN_POINT('Ctrl Pts',(0.297857995688647,-1.306435779838,2.90566182226115E-17));
#9995=CARTESIAN_POINT('',(0.9,-1.32024227787037,0.));
#9996=CARTESIAN_POINT('Ctrl Pts',(0.297857995688651,-1.306435779838,-5.81335652359571E-17));
#9997=CARTESIAN_POINT('Ctrl Pts',(0.498765834064439,-1.31101124067384,-1.02216845336465E-13));
#9998=CARTESIAN_POINT('Ctrl Pts',(0.699470314209512,-1.31560060357718,-4.73070532165219E-10));
#9999=CARTESIAN_POINT('Ctrl Pts',(0.9,-1.32024227787037,4.62320796019307E-17));
#10000=CARTESIAN_POINT('',(0.9,1.39290118819044,0.));
#10001=CARTESIAN_POINT('',(4.3,-1.41116952203211,0.));
#10002=CARTESIAN_POINT('Ctrl Pts',(1.10000000020724,-1.32489175811528,-9.82782277325449E-12));
#10003=CARTESIAN_POINT('Ctrl Pts',(2.16992692797068,-1.34987955410658,4.63225598025733E-9));
#10004=CARTESIAN_POINT('Ctrl Pts',(3.23514201430925,-1.37672428034078,3.20747301048384E-8));
#10005=CARTESIAN_POINT('Ctrl Pts',(4.3,-1.41116952203211,-8.74629427996717E-16));
#10006=CARTESIAN_POINT('',(4.3,1.48481481481482,0.));
#10007=CARTESIAN_POINT('',(8.7,-1.61160179736194,0.));
#10008=CARTESIAN_POINT('Ctrl Pts',(4.50000000001737,-1.41772989873549,-1.00870158580013E-12));
#10009=CARTESIAN_POINT('Ctrl Pts',(5.14541122039116,-1.43919849219739,1.84287460122322E-8));
#10010=CARTESIAN_POINT('Ctrl Pts',(5.79079200637672,-1.46358894290692,-2.29215846350395E-9));
#10011=CARTESIAN_POINT('Ctrl Pts',(6.43711407552466,-1.49221504703413,-7.12038357450289E-9));
#10012=CARTESIAN_POINT('Ctrl Pts',(6.48784335049204,-1.49446188584227,-7.49934689782436E-9));
#10013=CARTESIAN_POINT('Ctrl Pts',(6.5385784252675,-1.49673484630497,-7.6873350528488E-9));
#10014=CARTESIAN_POINT('Ctrl Pts',(6.58931977021612,-1.49903457911226,-7.60400982311631E-9));
#10015=CARTESIAN_POINT('Ctrl Pts',(7.29382172663923,-1.5309644828944,-6.44710735180711E-9));
#10016=CARTESIAN_POINT('Ctrl Pts',(7.99729122590638,-1.56795478022256,5.29179522587699E-9));
#10017=CARTESIAN_POINT('Ctrl Pts',(8.70000000002062,-1.61160179731554,-3.21479112539667E-13));
#10018=CARTESIAN_POINT('',(8.7,1.68851851851852,0.));
#10019=CARTESIAN_POINT('',(12.6,-1.93292824674167,0.));
#10020=CARTESIAN_POINT('',(12.8889963716306,-1.96391015057091,0.));
#10021=CARTESIAN_POINT('Ctrl Pts',(12.6000000004653,-1.93292824679067,-1.00288700954909E-16));
#10022=CARTESIAN_POINT('Ctrl Pts',(12.6963367945484,-1.94307238002033,2.28133307867826E-10));
#10023=CARTESIAN_POINT('Ctrl Pts',(12.7926686848896,-1.9533982851754,-5.07154825701885E-13));
#10024=CARTESIAN_POINT('Ctrl Pts',(12.8889963716306,-1.96391015057091,2.24786696790336E-16));
#10025=CARTESIAN_POINT('',(12.9997255308004,-1.86463850151065,-1.38777878078145E-17));
#10026=CARTESIAN_POINT('Ctrl Pts',(12.8889963716306,-1.96391015057091,5.29090660172926E-17));
#10027=CARTESIAN_POINT('Ctrl Pts',(12.8968843421745,-1.96477093437063,1.28387508960266E-11));
#10028=CARTESIAN_POINT('Ctrl Pts',(12.9048206871516,-1.96464841285931,-2.5989605143924E-6));
#10029=CARTESIAN_POINT('Ctrl Pts',(12.9126487282508,-1.9636130141884,-4.24292438262167E-6));
#10030=CARTESIAN_POINT('Ctrl Pts',(12.9176900487482,-1.96294620923983,-5.30165014054907E-6));
#10031=CARTESIAN_POINT('Ctrl Pts',(12.9226867577298,-1.96189962975099,-6.00943773338864E-6));
#10032=CARTESIAN_POINT('Ctrl Pts',(12.9275953864907,-1.96048085896027,-6.09358828708331E-6));
#10033=CARTESIAN_POINT('Ctrl Pts',(12.9352257743335,-1.95827540160737,-6.22439902734509E-6));
#10034=CARTESIAN_POINT('Ctrl Pts',(12.9425549137553,-1.95519874430406,-4.64402662178521E-6));
#10035=CARTESIAN_POINT('Ctrl Pts',(12.949425376669,-1.9513005478593,-3.15156624759025E-6));
#10036=CARTESIAN_POINT('Ctrl Pts',(12.9520760960011,-1.94979656991686,-2.57575445499556E-6));
#10037=CARTESIAN_POINT('Ctrl Pts',(12.9546583803074,-1.94816978416017,-2.04880625960079E-6));
#10038=CARTESIAN_POINT('Ctrl Pts',(12.9571622133441,-1.9464211898676,-1.82278374303809E-6));
#10039=CARTESIAN_POINT('Ctrl Pts',(12.9587955877505,-1.9452804951316,-1.67533805140214E-6));
#10040=CARTESIAN_POINT('Ctrl Pts',(12.9603955609302,-1.94408794089591,-1.65796127395168E-6));
#10041=CARTESIAN_POINT('Ctrl Pts',(12.9619602112942,-1.94284549575182,-1.70649031798611E-6));
#10042=CARTESIAN_POINT('Ctrl Pts',(12.9681665721336,-1.93791719798967,-1.89898620422551E-6));
#10043=CARTESIAN_POINT('Ctrl Pts',(12.9737470546445,-1.93226498850035,-2.8025064238469E-6));
#10044=CARTESIAN_POINT('Ctrl Pts',(12.9786034821464,-1.926037248212,-2.79230211737029E-6));
#10045=CARTESIAN_POINT('Ctrl Pts',(12.9817011960737,-1.92206483066456,-2.78579321297956E-6));
#10046=CARTESIAN_POINT('Ctrl Pts',(12.9845038017717,-1.91785723501915,-2.48811564693169E-6));
#10047=CARTESIAN_POINT('Ctrl Pts',(12.9869771252785,-1.91344616543364,-2.2918341012218E-6));
#10048=CARTESIAN_POINT('Ctrl Pts',(12.9874796596041,-1.91254991636901,-2.25195326317628E-6));
#10049=CARTESIAN_POINT('Ctrl Pts',(12.9879679417815,-1.9116463809131,-2.21866365029432E-6));
#10050=CARTESIAN_POINT('Ctrl Pts',(12.98844174868,-1.91073586520696,-2.19841011183313E-6));
#10051=CARTESIAN_POINT('Ctrl Pts',(12.9918929665356,-1.9041036526468,-2.05088297829219E-6));
#10052=CARTESIAN_POINT('Ctrl Pts',(12.9945793344589,-1.89710244289626,-2.35789128083535E-6));
#10053=CARTESIAN_POINT('Ctrl Pts',(12.9964698429198,-1.88986530397042,-1.93853625224654E-6));
#10054=CARTESIAN_POINT('Ctrl Pts',(12.9984668213505,-1.88222058265133,-1.49556391743615E-6));
#10055=CARTESIAN_POINT('Ctrl Pts',(12.9995610814633,-1.87437060764114,-2.4459616079733E-7));
#10056=CARTESIAN_POINT('Ctrl Pts',(12.9997084424383,-1.86646992060833,-2.60951667192209E-8));
#10057=CARTESIAN_POINT('Ctrl Pts',(12.9997198235207,-1.86585972940924,-9.21975031242219E-9));
#10058=CARTESIAN_POINT('Ctrl Pts',(12.9997255308031,-1.86524923282631,2.14479566203628E-13));
#10059=CARTESIAN_POINT('Ctrl Pts',(12.9997255308004,-1.86463850151065,-9.54097911787244E-18));
#10060=CARTESIAN_POINT('',(12.9997255308004,1.86463850151064,1.38777878078145E-17));
#10061=CARTESIAN_POINT('',(12.9997255308004,1.1,0.));
#10062=CARTESIAN_POINT('',(12.8889963716306,1.96391015057091,0.));
#10063=CARTESIAN_POINT('Ctrl Pts',(12.9997255308004,1.86463850151065,-9.97465998686664E-18));
#10064=CARTESIAN_POINT('Ctrl Pts',(12.9997255309996,1.87257112921612,1.42345874390777E-11));
#10065=CARTESIAN_POINT('Ctrl Pts',(12.9987425107347,1.88044501776258,-2.76622459581243E-6));
#10066=CARTESIAN_POINT('Ctrl Pts',(12.9968635501128,1.8881121101061,-4.50602169498049E-6));
#10067=CARTESIAN_POINT('Ctrl Pts',(12.9956551765012,1.89304287446485,-5.62489820561454E-6));
#10068=CARTESIAN_POINT('Ctrl Pts',(12.994075066483,1.89788828888188,-6.37205869803057E-6));
#10069=CARTESIAN_POINT('Ctrl Pts',(12.9921354490207,1.90260616696402,-6.45954116508302E-6));
#10070=CARTESIAN_POINT('Ctrl Pts',(12.9891151690915,1.90995262200289,-6.59576469602218E-6));
#10071=CARTESIAN_POINT('Ctrl Pts',(12.9852608829945,1.91690476599405,-4.92589918404109E-6));
#10072=CARTESIAN_POINT('Ctrl Pts',(12.9806393828366,1.92331154882078,-3.3382766296878E-6));
#10073=CARTESIAN_POINT('Ctrl Pts',(12.9788533632605,1.92578750666072,-2.72472586378502E-6));
#10074=CARTESIAN_POINT('Ctrl Pts',(12.9769522584487,1.92818179997524,-2.1610482659023E-6));
#10075=CARTESIAN_POINT('Ctrl Pts',(12.9749381758772,1.93048453804291,-1.90960564360578E-6));
#10076=CARTESIAN_POINT('Ctrl Pts',(12.9736352090466,1.93197424425657,-1.74694031832382E-6));
#10077=CARTESIAN_POINT('Ctrl Pts',(12.9722849384098,1.93342561524533,-1.71698229815602E-6));
#10078=CARTESIAN_POINT('Ctrl Pts',(12.9708894910408,1.9348369915754,-1.75552529092739E-6));
#10079=CARTESIAN_POINT('Ctrl Pts',(12.9653179015399,1.94047218048862,-1.90941553332435E-6));
#10080=CARTESIAN_POINT('Ctrl Pts',(12.9590944588136,1.94540670303376,-2.83773366290493E-6));
#10081=CARTESIAN_POINT('Ctrl Pts',(12.9523775255978,1.94955941520082,-2.8574013135715E-6));
#10082=CARTESIAN_POINT('Ctrl Pts',(12.9480923984168,1.95220867479748,-2.86994846593266E-6));
#10083=CARTESIAN_POINT('Ctrl Pts',(12.9436054681019,1.95453912223498,-2.59559485065602E-6));
#10084=CARTESIAN_POINT('Ctrl Pts',(12.9389519978263,1.95652032281755,-2.39773084743613E-6));
#10085=CARTESIAN_POINT('Ctrl Pts',(12.9379934875219,1.95692840561619,-2.35697530915642E-6));
#10086=CARTESIAN_POINT('Ctrl Pts',(12.9370291206935,1.95732112306527,-2.32193094846859E-6));
#10087=CARTESIAN_POINT('Ctrl Pts',(12.9360592398442,1.95769827921557,-2.29894501965994E-6));
#10088=CARTESIAN_POINT('Ctrl Pts',(12.929096105975,1.96040602292032,-2.13392052256244E-6));
#10089=CARTESIAN_POINT('Ctrl Pts',(12.9218497638689,1.96231496375013,-2.36509085467933E-6));
#10090=CARTESIAN_POINT('Ctrl Pts',(12.9144555496645,1.96340894166242,-1.92146179377921E-6));
#10091=CARTESIAN_POINT('Ctrl Pts',(12.9066371708262,1.96456567495722,-1.45238421961943E-6));
#10092=CARTESIAN_POINT('Ctrl Pts',(12.8987125532455,1.96480297730229,-2.37321368026999E-7));
#10093=CARTESIAN_POINT('Ctrl Pts',(12.8908401755085,1.96409377829808,-2.55627471131237E-8));
#10094=CARTESIAN_POINT('Ctrl Pts',(12.89022523009,1.96403837970149,-9.02136684357828E-9));
#10095=CARTESIAN_POINT('Ctrl Pts',(12.8896106033158,1.96397717928728,1.9621770460073E-13));
#10096=CARTESIAN_POINT('Ctrl Pts',(12.8889963716306,1.96391015057091,-3.29597460435593E-17));
#10097=CARTESIAN_POINT('',(12.6,1.93292824674167,0.));
#10098=CARTESIAN_POINT('Ctrl Pts',(12.8889963716306,1.96391015057091,8.95144418658345E-17));
#10099=CARTESIAN_POINT('Ctrl Pts',(12.7926686852738,1.95339828521733,-5.07275478770449E-13));
#10100=CARTESIAN_POINT('Ctrl Pts',(12.6963367949308,1.94307238006059,2.28132759158623E-10));
#10101=CARTESIAN_POINT('Ctrl Pts',(12.6000000004652,1.93292824679066,-1.5019386425618E-16));
#10102=CARTESIAN_POINT('',(12.6,-1.99376954809806,0.));
#10103=CARTESIAN_POINT('Origin',(11.2,0.,0.));
#10104=CARTESIAN_POINT('',(10.8,-4.89858719658942E-17,0.7));
#10105=CARTESIAN_POINT('Origin',(11.2,0.,0.7));
#10106=CARTESIAN_POINT('',(10.8,-4.89858719658942E-17,0.));
#10107=CARTESIAN_POINT('Origin',(2.,0.,0.));
#10108=CARTESIAN_POINT('',(1.6,-4.89858719658941E-17,0.));
#10109=CARTESIAN_POINT('Origin',(12.6,-1.99376954809806,0.));
#10110=CARTESIAN_POINT('',(12.6,-1.90428042248893,0.60470250816874));
#10111=CARTESIAN_POINT('Ctrl Pts',(12.6,-1.93292824674167,0.));
#10112=CARTESIAN_POINT('Ctrl Pts',(12.6,-1.92814118331811,0.100975624959503));
#10113=CARTESIAN_POINT('Ctrl Pts',(12.6,-1.9233557423333,0.20195205683881));
#10114=CARTESIAN_POINT('Ctrl Pts',(12.6,-1.91380649287245,0.40351907263528));
#10115=CARTESIAN_POINT('Ctrl Pts',(12.6,-1.90904260275794,0.504111110768618));
#10116=CARTESIAN_POINT('Ctrl Pts',(12.6,-1.90428042248893,0.60470250816874));
#10117=CARTESIAN_POINT('',(12.6,1.90428042248893,0.60470250816874));
#10118=CARTESIAN_POINT('Ctrl Pts',(12.6,1.90428042248893,0.60470250816874));
#10119=CARTESIAN_POINT('Ctrl Pts',(12.6,1.90904310126474,0.504100580823831));
#10120=CARTESIAN_POINT('Ctrl Pts',(12.6,1.91380749024866,0.403498012513773));
#10121=CARTESIAN_POINT('Ctrl Pts',(12.6,1.92335674041114,0.201930996640285));
#10122=CARTESIAN_POINT('Ctrl Pts',(12.6,1.92814168252712,0.100965094925255));
#10123=CARTESIAN_POINT('Ctrl Pts',(12.6,1.93292824674167,0.));
#10124=CARTESIAN_POINT('',(12.6,1.80383022254432,0.7));
#10125=CARTESIAN_POINT('Ctrl Pts',(12.6,1.80383022254432,0.7));
#10126=CARTESIAN_POINT('Ctrl Pts',(12.6,1.81177675668304,0.7));
#10127=CARTESIAN_POINT('Ctrl Pts',(12.6000021803669,1.81966206665253,0.699006623620781));
#10128=CARTESIAN_POINT('Ctrl Pts',(12.6000040789681,1.8273451885609,0.69711902809518));
#10129=CARTESIAN_POINT('Ctrl Pts',(12.6000050614635,1.8313210797205,0.696142227980247));
#10130=CARTESIAN_POINT('Ctrl Pts',(12.6000059683507,1.83524283435206,0.694925046992878));
#10131=CARTESIAN_POINT('Ctrl Pts',(12.6000066021136,1.83908960013903,0.693475985595303));
#10132=CARTESIAN_POINT('Ctrl Pts',(12.6000078338507,1.84656590463324,0.690659691378536));
#10133=CARTESIAN_POINT('Ctrl Pts',(12.6000078244032,1.85367932786264,0.687000939374075));
#10134=CARTESIAN_POINT('Ctrl Pts',(12.6000065509639,1.86028396908448,0.682580904467878));
#10135=CARTESIAN_POINT('Ctrl Pts',(12.600005740321,1.86448833536622,0.679767209507086));
#10136=CARTESIAN_POINT('Ctrl Pts',(12.6000044390918,1.86848632867783,0.676643963831362));
#10137=CARTESIAN_POINT('Ctrl Pts',(12.6000033339006,1.8722338275817,0.673223162566374));
#10138=CARTESIAN_POINT('Ctrl Pts',(12.6000024442799,1.87525036668517,0.670469597843409));
#10139=CARTESIAN_POINT('Ctrl Pts',(12.600001679327,1.8780865799519,0.667539409933064));
#10140=CARTESIAN_POINT('Ctrl Pts',(12.600001676908,1.88072259809992,0.664442334323256));
#10141=CARTESIAN_POINT('Ctrl Pts',(12.6000016722164,1.88583495965423,0.658435786041233));
#10142=CARTESIAN_POINT('Ctrl Pts',(12.6000042182276,1.89019731592974,0.651802923597933));
#10143=CARTESIAN_POINT('Ctrl Pts',(12.6000050838539,1.89374834224248,0.644708005294394));
#10144=CARTESIAN_POINT('Ctrl Pts',(12.60000518898,1.89417959722901,0.643846361750254));
#10145=CARTESIAN_POINT('Ctrl Pts',(12.6000052753339,1.8945988291305,0.642977876839351));
#10146=CARTESIAN_POINT('Ctrl Pts',(12.6000053405091,1.89500587920016,0.642102827114796));
#10147=CARTESIAN_POINT('Ctrl Pts',(12.6000058761205,1.89835102950234,0.634911640898031));
#10148=CARTESIAN_POINT('Ctrl Pts',(12.6000044960414,1.90083797337412,0.627363460372113));
#10149=CARTESIAN_POINT('Ctrl Pts',(12.6000025707297,1.90241244660326,0.619625605651968));
#10150=CARTESIAN_POINT('Ctrl Pts',(12.6000013488022,1.90341170938816,0.614714661398562));
#10151=CARTESIAN_POINT('Ctrl Pts',(12.5999999979477,1.90404256918024,0.609726685483646));
#10152=CARTESIAN_POINT('Ctrl Pts',(12.6000000000242,1.90428042250026,0.604702508168697));
#10153=CARTESIAN_POINT('',(12.6,-1.8038302225439,0.7));
#10154=CARTESIAN_POINT('',(12.6,-0.996884774049031,0.7));
#10155=CARTESIAN_POINT('Ctrl Pts',(12.6000000000242,-1.90428042250026,0.604702508168697));
#10156=CARTESIAN_POINT('Ctrl Pts',(12.5999999967566,-1.90390613686288,0.612608546261599));
#10157=CARTESIAN_POINT('Ctrl Pts',(12.6000030637542,-1.90256112855112,0.620429349781532));
#10158=CARTESIAN_POINT('Ctrl Pts',(12.6000044618611,-1.90032851942705,0.628004813168584));
#10159=CARTESIAN_POINT('Ctrl Pts',(12.6000051410147,-1.89924399238468,0.63168472059761));
#10160=CARTESIAN_POINT('Ctrl Pts',(12.6000055125137,-1.89794920179963,0.635306724151721));
#10161=CARTESIAN_POINT('Ctrl Pts',(12.6000054780251,-1.8964494555225,0.638851301608537));
#10162=CARTESIAN_POINT('Ctrl Pts',(12.6000054068101,-1.89335265044601,0.64617044994032));
#10163=CARTESIAN_POINT('Ctrl Pts',(12.6000033360581,-1.88942004582711,0.653077891556402));
#10164=CARTESIAN_POINT('Ctrl Pts',(12.6000021947065,-1.88472046879005,0.659412676045522));
#10165=CARTESIAN_POINT('Ctrl Pts',(12.6000018847951,-1.88344439178375,0.661132761228218));
#10166=CARTESIAN_POINT('Ctrl Pts',(12.6000016718208,-1.88211149822114,0.662810505670431));
#10167=CARTESIAN_POINT('Ctrl Pts',(12.6000016744967,-1.88072259784382,0.664442334323417));
#10168=CARTESIAN_POINT('Ctrl Pts',(12.6000016781594,-1.87882150924004,0.666675936463772));
#10169=CARTESIAN_POINT('Ctrl Pts',(12.6000020841502,-1.87681550570489,0.668823545630641));
#10170=CARTESIAN_POINT('Ctrl Pts',(12.6000026366798,-1.87471194035196,0.670881441794774));
#10171=CARTESIAN_POINT('Ctrl Pts',(12.6000041308351,-1.86902346102148,0.676446422116204));
#10172=CARTESIAN_POINT('Ctrl Pts',(12.600006461375,-1.86269053299793,0.681293522350018));
#10173=CARTESIAN_POINT('Ctrl Pts',(12.6000072160154,-1.85587841208407,0.685370830723365));
#10174=CARTESIAN_POINT('Ctrl Pts',(12.6000077023835,-1.85148797774957,0.687998669380522));
#10175=CARTESIAN_POINT('Ctrl Pts',(12.6000076405209,-1.84689749427555,0.690306084934615));
#10176=CARTESIAN_POINT('Ctrl Pts',(12.6000070464578,-1.84214500723865,0.692269637845719));
#10177=CARTESIAN_POINT('Ctrl Pts',(12.6000061272438,-1.8347913233911,0.69530790964196));
#10178=CARTESIAN_POINT('Ctrl Pts',(12.6000039197963,-1.82713360831075,0.697490862850871));
#10179=CARTESIAN_POINT('Ctrl Pts',(12.6000021173902,-1.81932000848244,0.698749700991972));
#10180=CARTESIAN_POINT('Ctrl Pts',(12.6000009388424,-1.81421089282246,0.699572823470905));
#10181=CARTESIAN_POINT('Ctrl Pts',(12.6,-1.80903450780073,0.7));
#10182=CARTESIAN_POINT('Ctrl Pts',(12.6,-1.80383022254432,0.7));
#10183=CARTESIAN_POINT('Ctrl Pts',(12.4277899437912,-1.91498765980368,8.1061082099175E-6));
#10184=CARTESIAN_POINT('Ctrl Pts',(12.4185093097394,-1.90440735427916,0.201956437811591));
#10185=CARTESIAN_POINT('Ctrl Pts',(12.4092288296506,-1.89382707230216,0.403904777849331));
#10186=CARTESIAN_POINT('Ctrl Pts',(12.3999485057213,-1.88324681432718,0.605853126346544));
#10187=CARTESIAN_POINT('Ctrl Pts',(11.2514531524596,-1.79377193015415,-0.000335869645892519));
#10188=CARTESIAN_POINT('Ctrl Pts',(11.2440495594319,-1.78319067664719,0.201611894978303));
#10189=CARTESIAN_POINT('Ctrl Pts',(11.2366461029568,-1.77260943823668,0.403559665746509));
#10190=CARTESIAN_POINT('Ctrl Pts',(11.2292427771396,-1.76202821861547,0.605507441576721));
#10191=CARTESIAN_POINT('Ctrl Pts',(10.0755218259154,-1.69940246002113,-0.00057195363688788));
#10192=CARTESIAN_POINT('Ctrl Pts',(10.0699958446785,-1.68882059084335,0.201375418496625));
#10193=CARTESIAN_POINT('Ctrl Pts',(10.0644699805481,-1.67823873210945,0.403322794723726));
#10194=CARTESIAN_POINT('Ctrl Pts',(10.0589442279885,-1.66765688783508,0.605270174140068));
#10195=CARTESIAN_POINT('Ctrl Pts',(8.90001330805802,-1.62424530699552,-0.000736768987564917));
#10196=CARTESIAN_POINT('Ctrl Pts',(8.89636559238287,-1.61366301035882,0.201210329036737));
#10197=CARTESIAN_POINT('Ctrl Pts',(8.89271797406169,-1.60308072296431,0.403157429313698));
#10198=CARTESIAN_POINT('Ctrl Pts',(8.88907045450167,-1.59249844499155,0.605104531878289));
#10199=CARTESIAN_POINT('Ctrl Pts',(8.9000000009702,-1.5932011715731,0.605106081469384));
#10200=CARTESIAN_POINT('Ctrl Pts',(10.0684994345535,-1.66840362346204,0.605023135335662));
#10201=CARTESIAN_POINT('Ctrl Pts',(11.2356615742313,-1.76272273105624,0.604904457271936));
#10202=CARTESIAN_POINT('Ctrl Pts',(12.4,-1.8833055216247,0.604732563714112));
#10203=CARTESIAN_POINT('Ctrl Pts',(12.8889963716306,-1.96391015057091,2.25514051876985E-16));
#10204=CARTESIAN_POINT('Ctrl Pts',(12.8789974396847,-1.95334878321431,0.201594505485581));
#10205=CARTESIAN_POINT('Ctrl Pts',(12.8689986695879,-1.94278744208821,0.403189020401051));
#10206=CARTESIAN_POINT('Ctrl Pts',(12.8590000636394,-1.93222612769726,0.604783544887274));
#10207=CARTESIAN_POINT('Ctrl Pts',(12.792662965057,-1.95339909479377,-3.05216148415599E-5));
#10208=CARTESIAN_POINT('Ctrl Pts',(12.7828174539371,-1.94283764251598,0.201563933758495));
#10209=CARTESIAN_POINT('Ctrl Pts',(12.7729721028852,-1.93227621586528,0.403158398317997));
#10210=CARTESIAN_POINT('Ctrl Pts',(12.7631269141758,-1.92171481533493,0.604752872200892));
#10211=CARTESIAN_POINT('Ctrl Pts',(12.6963322449993,-1.94307475200589,-6.02899321993968E-5));
#10212=CARTESIAN_POINT('Ctrl Pts',(12.6866401583647,-1.93251321719056,0.201534116532542));
#10213=CARTESIAN_POINT('Ctrl Pts',(12.6769482300299,-1.92195170741534,0.403128531945268));
#10214=CARTESIAN_POINT('Ctrl Pts',(12.6672564622455,-1.91139022316239,0.604722956439736));
#10215=CARTESIAN_POINT('Ctrl Pts',(12.6000042264769,-1.9329329264796,-8.93242901516475E-5));
#10216=CARTESIAN_POINT('Ctrl Pts',(12.5904655680581,-1.92237131142302,0.201505034443145));
#10217=CARTESIAN_POINT('Ctrl Pts',(12.5809270661843,-1.91180972083551,0.403099401891705));
#10218=CARTESIAN_POINT('Ctrl Pts',(12.5713887230828,-1.90124815518829,0.604693778185974));
#10219=CARTESIAN_POINT('',(12.8572578715866,-1.93204080633595,0.60466226999893));
#10220=CARTESIAN_POINT('Ctrl Pts',(12.6000000000242,-1.90428042250026,0.604702508168697));
#10221=CARTESIAN_POINT('Ctrl Pts',(12.6857696261193,-1.91338852735451,0.604689390578107));
#10222=CARTESIAN_POINT('Ctrl Pts',(12.7715225733429,-1.92264108900731,0.604675979983877));
#10223=CARTESIAN_POINT('Ctrl Pts',(12.8572578715866,-1.93204080633595,0.60466226999893));
#10224=CARTESIAN_POINT('Ctrl Pts',(12.8572578715866,-1.93204080633595,0.604662269998931));
#10225=CARTESIAN_POINT('Ctrl Pts',(12.867837444884,-1.94266422047353,0.403108198925376));
#10226=CARTESIAN_POINT('Ctrl Pts',(12.8784169445746,-1.95328733374019,0.201554108835025));
#10227=CARTESIAN_POINT('Ctrl Pts',(12.8889963716306,-1.96391015057091,-1.13624387676481E-16));
#10228=CARTESIAN_POINT('Ctrl Pts',(12.4102890066107,-1.7839488953552,0.7));
#10229=CARTESIAN_POINT('Ctrl Pts',(11.2423261062923,-1.6629989551888,0.7));
#10230=CARTESIAN_POINT('Ctrl Pts',(10.0717272052363,-1.56846077660453,0.7));
#10231=CARTESIAN_POINT('Ctrl Pts',(8.89999999999993,-1.49312521822106,0.7));
#10232=CARTESIAN_POINT('Ctrl Pts',(12.4072999778185,-1.81281269415102,0.7));
#10233=CARTESIAN_POINT('Ctrl Pts',(11.2397765858669,-1.69187462084457,0.699998757165067));
#10234=CARTESIAN_POINT('Ctrl Pts',(10.0695527221263,-1.59734372851255,0.700000594792869));
#10235=CARTESIAN_POINT('Ctrl Pts',(8.89814271406455,-1.52201240649035,0.7));
#10236=CARTESIAN_POINT('Ctrl Pts',(12.4021203845267,-1.86282985658401,0.676448561733929));
#10237=CARTESIAN_POINT('Ctrl Pts',(11.2353531757414,-1.74191593276004,0.676505236381959));
#10238=CARTESIAN_POINT('Ctrl Pts',(10.0657879841113,-1.64739716848489,0.676543604639643));
#10239=CARTESIAN_POINT('Ctrl Pts',(8.89492397206972,-1.57207492202614,0.676570833338327));
#10240=CARTESIAN_POINT('Ctrl Pts',(12.400106093269,-1.88228102337346,0.626471792264191));
#10241=CARTESIAN_POINT('Ctrl Pts',(11.2336287644773,-1.76143987438699,0.626617923584012));
#10242=CARTESIAN_POINT('Ctrl Pts',(10.0643137348541,-1.66697079985262,0.626717999675944));
#10243=CARTESIAN_POINT('Ctrl Pts',(8.89366330605793,-1.59168261717615,0.626788336025017));
#10244=CARTESIAN_POINT('Ctrl Pts',(12.4,-1.8833055216247,0.604732563714112));
#10245=CARTESIAN_POINT('Ctrl Pts',(11.2335332423564,-1.7625023138725,0.604904771481731));
#10246=CARTESIAN_POINT('Ctrl Pts',(10.0642324382527,-1.66805889332185,0.605023569028795));
#10247=CARTESIAN_POINT('Ctrl Pts',(8.89359217382714,-1.59278896817116,0.605106535971077));
#10248=CARTESIAN_POINT('Ctrl Pts',(12.400000003046,-1.78288409409898,0.7));
#10249=CARTESIAN_POINT('Ctrl Pts',(11.235451325406,-1.66244391065713,0.7));
#10250=CARTESIAN_POINT('Ctrl Pts',(10.0682865064676,-1.56823955876321,0.7));
#10251=CARTESIAN_POINT('Ctrl Pts',(8.89999999999993,-1.49312521822106,0.7));
#10252=CARTESIAN_POINT('Ctrl Pts',(12.8681436286308,-1.83274446434879,0.7));
#10253=CARTESIAN_POINT('Ctrl Pts',(12.7787800350189,-1.82294762441299,0.7));
#10254=CARTESIAN_POINT('Ctrl Pts',(12.6893984576578,-1.8133105623702,0.7));
#10255=CARTESIAN_POINT('Ctrl Pts',(12.6,-1.80383022254431,0.7));
#10256=CARTESIAN_POINT('Ctrl Pts',(12.8649798835675,-1.86160311979107,0.7));
#10257=CARTESIAN_POINT('Ctrl Pts',(12.7756511334299,-1.85180730951691,0.699999896874207));
#10258=CARTESIAN_POINT('Ctrl Pts',(12.686303642571,-1.84217134991284,0.700000098415946));
#10259=CARTESIAN_POINT('Ctrl Pts',(12.5969393303221,-1.83269196733649,0.7));
#10260=CARTESIAN_POINT('Ctrl Pts',(12.8594976525144,-1.91161025179704,0.676425356750174));
#10261=CARTESIAN_POINT('Ctrl Pts',(12.7702288461641,-1.90181652272411,0.676430055978541));
#10262=CARTESIAN_POINT('Ctrl Pts',(12.6809412203008,-1.89218243450198,0.676434576658958));
#10263=CARTESIAN_POINT('Ctrl Pts',(12.5916356538948,-1.88270499442535,0.67643906321291));
#10264=CARTESIAN_POINT('Ctrl Pts',(12.8573684983393,-1.93103170500986,0.626412260100396));
#10265=CARTESIAN_POINT('Ctrl Pts',(12.7681225846323,-1.92124403769089,0.626424372515079));
#10266=CARTESIAN_POINT('Ctrl Pts',(12.6788572782757,-1.91161594713487,0.626436135819418));
#10267=CARTESIAN_POINT('Ctrl Pts',(12.5895741974899,-1.90214427893475,0.626447702441804));
#10268=CARTESIAN_POINT('Ctrl Pts',(12.8572578715866,-1.93204080633595,0.60466226999893));
#10269=CARTESIAN_POINT('Ctrl Pts',(12.7680127446979,-1.92225628370762,0.604676541242762));
#10270=CARTESIAN_POINT('Ctrl Pts',(12.6787484942245,-1.91263121188365,0.60469048808123));
#10271=CARTESIAN_POINT('Ctrl Pts',(12.5894662143615,-1.9031625467727,0.604704117718382));
#10272=CARTESIAN_POINT('',(12.8681436286308,-1.83274446434879,0.7));
#10273=CARTESIAN_POINT('Ctrl Pts',(12.8681436286308,-1.83274446434879,0.7));
#10274=CARTESIAN_POINT('Ctrl Pts',(12.7787800350189,-1.82294762441299,0.7));
#10275=CARTESIAN_POINT('Ctrl Pts',(12.6893984576578,-1.8133105623702,0.7));
#10276=CARTESIAN_POINT('Ctrl Pts',(12.6,-1.80383022254431,0.7));
#10277=CARTESIAN_POINT('Origin',(12.8681436286308,-1.83274446434879,0.6));
#10278=CARTESIAN_POINT('Origin',(6.87409734069396,-2.22251806091942E-16,
0.7));
#10279=CARTESIAN_POINT('Ctrl Pts',(8.9,1.49312521822106,0.7));
#10280=CARTESIAN_POINT('Ctrl Pts',(10.0682865064677,1.56823955876321,0.7));
#10281=CARTESIAN_POINT('Ctrl Pts',(11.2354513254061,1.66244391065714,0.7));
#10282=CARTESIAN_POINT('Ctrl Pts',(12.4000000030461,1.78288409409899,0.7));
#10283=CARTESIAN_POINT('Origin',(6.87409734069396,-2.22251806091942E-16,
0.7));
#10284=CARTESIAN_POINT('',(12.8681436286308,1.83274446434879,0.7));
#10285=CARTESIAN_POINT('Ctrl Pts',(12.6,1.80383022254432,0.7));
#10286=CARTESIAN_POINT('Ctrl Pts',(12.6893984576578,1.8133105623702,0.7));
#10287=CARTESIAN_POINT('Ctrl Pts',(12.7787800350189,1.82294762441299,0.7));
#10288=CARTESIAN_POINT('Ctrl Pts',(12.8681436286308,1.83274446434879,0.7));
#10289=CARTESIAN_POINT('',(12.8681436286308,1.1,0.7));
#10290=CARTESIAN_POINT('Ctrl Pts',(8.9,1.49312521822106,0.7));
#10291=CARTESIAN_POINT('Ctrl Pts',(10.0717272052363,1.56846077660453,0.7));
#10292=CARTESIAN_POINT('Ctrl Pts',(11.2423261062923,1.6629989551888,0.7));
#10293=CARTESIAN_POINT('Ctrl Pts',(12.4102890066107,1.7839488953552,0.7));
#10294=CARTESIAN_POINT('Ctrl Pts',(8.89814271406461,1.52201240649035,0.7));
#10295=CARTESIAN_POINT('Ctrl Pts',(10.0695527221263,1.59734372851256,0.700000594792869));
#10296=CARTESIAN_POINT('Ctrl Pts',(11.2397765858669,1.69187462084457,0.699998757165067));
#10297=CARTESIAN_POINT('Ctrl Pts',(12.4072999778185,1.81281269415102,0.7));
#10298=CARTESIAN_POINT('Ctrl Pts',(8.89492397206979,1.57207492202615,0.676570833338327));
#10299=CARTESIAN_POINT('Ctrl Pts',(10.0657879841114,1.64739716848489,0.676543604639644));
#10300=CARTESIAN_POINT('Ctrl Pts',(11.2353531757414,1.74191593276004,0.676505236381959));
#10301=CARTESIAN_POINT('Ctrl Pts',(12.4021203845267,1.86282985658401,0.676448561733929));
#10302=CARTESIAN_POINT('Ctrl Pts',(8.89366330605799,1.59168261717616,0.626788336025017));
#10303=CARTESIAN_POINT('Ctrl Pts',(10.0643137348542,1.66697079985262,0.626717999675944));
#10304=CARTESIAN_POINT('Ctrl Pts',(11.2336287644773,1.761439874387,0.626617923584012));
#10305=CARTESIAN_POINT('Ctrl Pts',(12.400106093269,1.88228102337346,0.626471792264191));
#10306=CARTESIAN_POINT('Ctrl Pts',(8.89359217382721,1.59278896817116,0.605106535971077));
#10307=CARTESIAN_POINT('Ctrl Pts',(10.0642324382527,1.66805889332185,0.605023569028795));
#10308=CARTESIAN_POINT('Ctrl Pts',(11.2335332423565,1.7625023138725,0.604904771481731));
#10309=CARTESIAN_POINT('Ctrl Pts',(12.4,1.8833055216247,0.604732563714112));
#10310=CARTESIAN_POINT('Ctrl Pts',(12.4,1.8833055216247,0.604732563714112));
#10311=CARTESIAN_POINT('Ctrl Pts',(11.2356615742313,1.76272273105624,0.604904457271936));
#10312=CARTESIAN_POINT('Ctrl Pts',(10.0684994345535,1.66840362346204,0.605023135335662));
#10313=CARTESIAN_POINT('Ctrl Pts',(8.90000000097019,1.5932011715731,0.605106081469384));
#10314=CARTESIAN_POINT('Ctrl Pts',(8.90001330805765,1.62424530699444,-0.000736768966955875));
#10315=CARTESIAN_POINT('Ctrl Pts',(8.89636559238262,1.6136630103581,0.201210329050476));
#10316=CARTESIAN_POINT('Ctrl Pts',(8.89271797406156,1.60308072296395,0.403157429320568));
#10317=CARTESIAN_POINT('Ctrl Pts',(8.88907045450167,1.59249844499155,0.605104531878289));
#10318=CARTESIAN_POINT('Ctrl Pts',(10.0755218259151,1.69940246002007,-0.000571953616278766));
#10319=CARTESIAN_POINT('Ctrl Pts',(10.0699958446785,1.68882059084265,0.201375418510364));
#10320=CARTESIAN_POINT('Ctrl Pts',(10.0644699805483,1.67823873210911,0.403322794730596));
#10321=CARTESIAN_POINT('Ctrl Pts',(10.0589442279888,1.6676568878351,0.605270174140069));
#10322=CARTESIAN_POINT('Ctrl Pts',(11.2514531524595,1.79377193015312,-0.000335869625283423));
#10323=CARTESIAN_POINT('Ctrl Pts',(11.244049559432,1.78319067664652,0.201611894992042));
#10324=CARTESIAN_POINT('Ctrl Pts',(11.2366461029572,1.77260943823637,0.403559665753379));
#10325=CARTESIAN_POINT('Ctrl Pts',(11.2292427771402,1.76202821861552,0.605507441576721));
#10326=CARTESIAN_POINT('Ctrl Pts',(12.4277899437912,1.9149876598027,8.10612881915578E-6));
#10327=CARTESIAN_POINT('Ctrl Pts',(12.4185093097397,1.90440735427854,0.201956437825331));
#10328=CARTESIAN_POINT('Ctrl Pts',(12.4092288296513,1.89382707230189,0.403904777856201));
#10329=CARTESIAN_POINT('Ctrl Pts',(12.3999485057223,1.88324681432728,0.605853126346545));
#10330=CARTESIAN_POINT('Ctrl Pts',(12.6000042264759,1.9329329264795,-8.93242901520291E-5));
#10331=CARTESIAN_POINT('Ctrl Pts',(12.5904655680574,1.92237131142328,0.201505034436202));
#10332=CARTESIAN_POINT('Ctrl Pts',(12.580927066184,1.91180972083614,0.403099401877819));
#10333=CARTESIAN_POINT('Ctrl Pts',(12.5713887230828,1.90124815518927,0.604693778165146));
#10334=CARTESIAN_POINT('Ctrl Pts',(12.6963322449987,1.94307475200582,-6.02899321996874E-5));
#10335=CARTESIAN_POINT('Ctrl Pts',(12.6866401583644,1.93251321719085,0.201534116525599));
#10336=CARTESIAN_POINT('Ctrl Pts',(12.6769482300299,1.921951707416,0.403128531931383));
#10337=CARTESIAN_POINT('Ctrl Pts',(12.6672564622458,1.91139022316341,0.604722956418908));
#10338=CARTESIAN_POINT('Ctrl Pts',(12.7926629650567,1.95339909479374,-3.05216148420481E-5));
#10339=CARTESIAN_POINT('Ctrl Pts',(12.7828174539371,1.94283764251631,0.201563933751552));
#10340=CARTESIAN_POINT('Ctrl Pts',(12.7729721028855,1.93227621586597,0.403158398304112));
#10341=CARTESIAN_POINT('Ctrl Pts',(12.7631269141765,1.92171481533599,0.604752872180064));
#10342=CARTESIAN_POINT('Ctrl Pts',(12.8889963716306,1.96391015057091,-1.66533453693773E-16));
#10343=CARTESIAN_POINT('Ctrl Pts',(12.878997439685,1.95334878321468,0.201594505478638));
#10344=CARTESIAN_POINT('Ctrl Pts',(12.8689986695886,1.94278744208894,0.403189020387166));
#10345=CARTESIAN_POINT('Ctrl Pts',(12.8590000636404,1.93222612769835,0.604783544866446));
#10346=CARTESIAN_POINT('',(12.8572578715866,1.93204080633595,0.60466226999893));
#10347=CARTESIAN_POINT('Ctrl Pts',(12.8889963716306,1.96391015057091,-3.88144377749811E-17));
#10348=CARTESIAN_POINT('Ctrl Pts',(12.8784169445746,1.95328733374019,0.201554108835021));
#10349=CARTESIAN_POINT('Ctrl Pts',(12.867837444884,1.94266422047353,0.403108198925375));
#10350=CARTESIAN_POINT('Ctrl Pts',(12.8572578715866,1.93204080633595,0.604662269998929));
#10351=CARTESIAN_POINT('Ctrl Pts',(12.8572578715866,1.93204080633595,0.60466226999893));
#10352=CARTESIAN_POINT('Ctrl Pts',(12.7715225733429,1.92264108900731,0.604675979983877));
#10353=CARTESIAN_POINT('Ctrl Pts',(12.6857696261193,1.91338852735451,0.604689390578107));
#10354=CARTESIAN_POINT('Ctrl Pts',(12.6000000000242,1.90428042250026,0.604702508168697));
#10355=CARTESIAN_POINT('Origin',(8.7,1.68851851851852,0.));
#10356=CARTESIAN_POINT('',(8.7,-1.5805153611151,0.605119933308333));
#10357=CARTESIAN_POINT('Ctrl Pts',(8.7,-1.5805153611151,0.605119933308333));
#10358=CARTESIAN_POINT('Ctrl Pts',(8.7,-1.58569938832865,0.504197823486131));
#10359=CARTESIAN_POINT('Ctrl Pts',(8.7,-1.59088373519313,0.403275164205241));
#10360=CARTESIAN_POINT('Ctrl Pts',(8.7,-1.60124586355191,0.201568897935389));
#10361=CARTESIAN_POINT('Ctrl Pts',(8.7,-1.60642370224807,0.10078416210737));
#10362=CARTESIAN_POINT('Ctrl Pts',(8.7,-1.61160179736194,0.));
#10363=CARTESIAN_POINT('',(8.7,-1.48045180431786,0.7));
#10364=CARTESIAN_POINT('Ctrl Pts',(8.70000000036779,-1.48045180452391,0.7));
#10365=CARTESIAN_POINT('Ctrl Pts',(8.70000000202598,-1.48836706478042,0.699999999180279));
#10366=CARTESIAN_POINT('Ctrl Pts',(8.70000127066624,-1.49622113223642,0.699007614827928));
#10367=CARTESIAN_POINT('Ctrl Pts',(8.70000237141531,-1.50387364922569,0.697121884028934));
#10368=CARTESIAN_POINT('Ctrl Pts',(8.70000291188189,-1.50763102664002,0.696195992283305));
#10369=CARTESIAN_POINT('Ctrl Pts',(8.70000341240591,-1.51133980954515,0.695053883793301));
#10370=CARTESIAN_POINT('Ctrl Pts',(8.70000377175886,-1.51498230649063,0.693702880475192));
#10371=CARTESIAN_POINT('Ctrl Pts',(8.70000450976793,-1.52246296255016,0.690928302676144));
#10372=CARTESIAN_POINT('Ctrl Pts',(8.70000452394134,-1.52958344744078,0.687306123577328));
#10373=CARTESIAN_POINT('Ctrl Pts',(8.70000379461986,-1.53619834892264,0.682919715776694));
#10374=CARTESIAN_POINT('Ctrl Pts',(8.70000333219987,-1.54039247012311,0.680138551763745));
#10375=CARTESIAN_POINT('Ctrl Pts',(8.70000258238552,-1.54438316197938,0.67704909562189));
#10376=CARTESIAN_POINT('Ctrl Pts',(8.70000192913237,-1.54812716280968,0.67366362845569));
#10377=CARTESIAN_POINT('Ctrl Pts',(8.70000138361353,-1.55125370412533,0.670836491537814));
#10378=CARTESIAN_POINT('Ctrl Pts',(8.70000090341281,-1.55418891097064,0.66782012731024));
#10379=CARTESIAN_POINT('Ctrl Pts',(8.7000009033621,-1.55691103280728,0.664625500020687));
#10380=CARTESIAN_POINT('Ctrl Pts',(8.7000009032669,-1.56202159382457,0.658627848677152));
#10381=CARTESIAN_POINT('Ctrl Pts',(8.70000241148087,-1.56638404855443,0.652003279246098));
#10382=CARTESIAN_POINT('Ctrl Pts',(8.70000292788623,-1.5699383402149,0.64491699469699));
#10383=CARTESIAN_POINT('Ctrl Pts',(8.70000298354275,-1.57032141040405,0.644153257609021));
#10384=CARTESIAN_POINT('Ctrl Pts',(8.70000303046442,-1.57069504840788,0.643384135640712));
#10385=CARTESIAN_POINT('Ctrl Pts',(8.70000306761332,-1.57105914547653,0.642609822781892));
#10386=CARTESIAN_POINT('Ctrl Pts',(8.70000341208914,-1.57443535963509,0.635429742901602));
#10387=CARTESIAN_POINT('Ctrl Pts',(8.70000263566904,-1.57695592401075,0.627888404173009));
#10388=CARTESIAN_POINT('Ctrl Pts',(8.70000151703179,-1.57856725066757,0.620153930269154));
#10389=CARTESIAN_POINT('Ctrl Pts',(8.70000080174396,-1.57959757782623,0.615208292159515));
#10390=CARTESIAN_POINT('Ctrl Pts',(8.7,-1.58025528705454,0.610183028431161));
#10391=CARTESIAN_POINT('Ctrl Pts',(8.7,-1.5805153611151,0.605119933308333));
#10392=CARTESIAN_POINT('',(8.7,1.48045180431904,0.7));
#10393=CARTESIAN_POINT('',(8.7,0.844259259259259,0.7));
#10394=CARTESIAN_POINT('',(8.7,1.5805153611151,0.605119933308333));
#10395=CARTESIAN_POINT('Ctrl Pts',(8.7,1.5805153611151,0.605119933308333));
#10396=CARTESIAN_POINT('Ctrl Pts',(8.7,1.58010890623597,0.61303275518587));
#10397=CARTESIAN_POINT('Ctrl Pts',(8.70000179355525,1.57873376841273,0.620855553142259));
#10398=CARTESIAN_POINT('Ctrl Pts',(8.7000025961206,1.5764741717406,0.62842799710221));
#10399=CARTESIAN_POINT('Ctrl Pts',(8.70000304562639,1.57520860278123,0.632669218617747));
#10400=CARTESIAN_POINT('Ctrl Pts',(8.70000324668712,1.57366457852079,0.636831947144834));
#10401=CARTESIAN_POINT('Ctrl Pts',(8.70000313318341,1.57185009366145,0.640886032861668));
#10402=CARTESIAN_POINT('Ctrl Pts',(8.70000293045856,1.56860930815545,0.648126888117959));
#10403=CARTESIAN_POINT('Ctrl Pts',(8.70000158438082,1.56454425420738,0.654942317779106));
#10404=CARTESIAN_POINT('Ctrl Pts',(8.70000106269264,1.55971945710293,0.661169479919421));
#10405=CARTESIAN_POINT('Ctrl Pts',(8.70000096439252,1.55881033523018,0.662342845179011));
#10406=CARTESIAN_POINT('Ctrl Pts',(8.70000090351839,1.55787410801649,0.663495254390581));
#10407=CARTESIAN_POINT('Ctrl Pts',(8.70000090409683,1.55691103285321,0.664625500020665));
#10408=CARTESIAN_POINT('Ctrl Pts',(8.70000090523835,1.55501044337284,0.666855993586132));
#10409=CARTESIAN_POINT('Ctrl Pts',(8.70000114361209,1.55300532702719,0.669000219206223));
#10410=CARTESIAN_POINT('Ctrl Pts',(8.70000146777886,1.55090303951829,0.671054438207787));
#10411=CARTESIAN_POINT('Ctrl Pts',(8.70000234447876,1.54521746205001,0.676610015749294));
#10412=CARTESIAN_POINT('Ctrl Pts',(8.70000370702799,1.53888821826629,0.681447385411957));
#10413=CARTESIAN_POINT('Ctrl Pts',(8.70000415375638,1.53207947242364,0.685512859850771));
#10414=CARTESIAN_POINT('Ctrl Pts',(8.70000443876751,1.52773551673798,0.688106618115728));
#10415=CARTESIAN_POINT('Ctrl Pts',(8.70000441165582,1.52319541573235,0.690385508075002));
#10416=CARTESIAN_POINT('Ctrl Pts',(8.70000407315693,1.51849599021366,0.692326230693156));
#10417=CARTESIAN_POINT('Ctrl Pts',(8.70000354533424,1.51116815716702,0.695352407250086));
#10418=CARTESIAN_POINT('Ctrl Pts',(8.70000225790696,1.50353761203248,0.697524030080351));
#10419=CARTESIAN_POINT('Ctrl Pts',(8.70000121423997,1.49575164755759,0.698771658000832));
#10420=CARTESIAN_POINT('Ctrl Pts',(8.70000053774506,1.49070486028667,0.699580358416591));
#10421=CARTESIAN_POINT('Ctrl Pts',(8.70000000144466,1.48559217323052,0.699999999467653));
#10422=CARTESIAN_POINT('Ctrl Pts',(8.70000000036779,1.48045180452391,0.7));
#10423=CARTESIAN_POINT('Ctrl Pts',(8.7,1.61160179736194,0.));
#10424=CARTESIAN_POINT('Ctrl Pts',(8.7,1.60642368739695,0.100784451162898));
#10425=CARTESIAN_POINT('Ctrl Pts',(8.7,1.60124583384883,0.201569476094892));
#10426=CARTESIAN_POINT('Ctrl Pts',(8.7,1.59088370548997,0.403275742430776));
#10427=CARTESIAN_POINT('Ctrl Pts',(8.7,1.58569937347746,0.504198112607714));
#10428=CARTESIAN_POINT('Ctrl Pts',(8.7,1.5805153611151,0.605119933308333));
#10429=CARTESIAN_POINT('Ctrl Pts',(8.7100201910492,-1.61222456240079,1.33887903992595E-6));
#10430=CARTESIAN_POINT('Ctrl Pts',(8.70667727354472,-1.60164608969543,0.201874135619687));
#10431=CARTESIAN_POINT('Ctrl Pts',(8.70333445073708,-1.59106762573893,0.40374693439627));
#10432=CARTESIAN_POINT('Ctrl Pts',(8.69999172399519,-1.58048917070122,0.605619735240497));
#10433=CARTESIAN_POINT('Ctrl Pts',(7.30266630830786,-1.52469223633113,-0.000186944012493601));
#10434=CARTESIAN_POINT('Ctrl Pts',(7.3015714609838,-1.51411327886182,0.201685539385837));
#10435=CARTESIAN_POINT('Ctrl Pts',(7.30047669312962,-1.50353432123569,0.403558023359813));
#10436=CARTESIAN_POINT('Ctrl Pts',(7.2993819983171,-1.49295537435081,0.605430507723141));
#10437=CARTESIAN_POINT('Ctrl Pts',(5.89591889571946,-1.46411055243784,-0.000276130330627546));
#10438=CARTESIAN_POINT('Ctrl Pts',(5.8970730573458,-1.45353136553189,0.201596203763285));
#10439=CARTESIAN_POINT('Ctrl Pts',(5.89822728315403,-1.44295217665945,0.403468537584815));
#10440=CARTESIAN_POINT('Ctrl Pts',(5.89938156763751,-1.43237299696387,0.60534087113472));
#10441=CARTESIAN_POINT('Ctrl Pts',(4.48978738186403,-1.41740792524342,-0.000330195618103912));
#10442=CARTESIAN_POINT('Ctrl Pts',(4.49319153668887,-1.4068286019831,0.201542048187911));
#10443=CARTESIAN_POINT('Ctrl Pts',(4.49659574248722,-1.39624928130228,0.403414291272231));
#10444=CARTESIAN_POINT('Ctrl Pts',(4.5,-1.3856699632509,0.605286533625018));
#10445=CARTESIAN_POINT('Ctrl Pts',(4.50000000014037,-1.38566996330298,0.605286533623957));
#10446=CARTESIAN_POINT('Ctrl Pts',(5.90109530155974,-1.43243455365708,0.605259331490037));
#10447=CARTESIAN_POINT('Ctrl Pts',(7.30150776148394,-1.49309969195427,0.605214402664297));
#10448=CARTESIAN_POINT('Ctrl Pts',(8.7,-1.5805153611151,0.605119933308333));
#10449=CARTESIAN_POINT('Ctrl Pts',(8.7062300060629,-1.48084102486261,0.7));
#10450=CARTESIAN_POINT('Ctrl Pts',(7.30535837857749,-1.39328148786737,0.7));
#10451=CARTESIAN_POINT('Ctrl Pts',(5.90286553803659,-1.3325543763676,0.7));
#10452=CARTESIAN_POINT('Ctrl Pts',(4.5,-1.28575421950843,0.7));
#10453=CARTESIAN_POINT('Ctrl Pts',(8.7044244076592,-1.50972892972339,0.7));
#10454=CARTESIAN_POINT('Ctrl Pts',(7.30392377861185,-1.42217417124324,0.699999322371676));
#10455=CARTESIAN_POINT('Ctrl Pts',(5.90170976758769,-1.36144968116949,0.700000194339816));
#10456=CARTESIAN_POINT('Ctrl Pts',(4.49903600403804,-1.314650633636,0.7));
#10457=CARTESIAN_POINT('Ctrl Pts',(8.70129509098077,-1.55979510296572,0.676577193851887));
#10458=CARTESIAN_POINT('Ctrl Pts',(7.30143307762773,-1.47225060169427,0.676608218952397));
#10459=CARTESIAN_POINT('Ctrl Pts',(5.89970879741633,-1.41153023905743,0.676622651488038));
#10460=CARTESIAN_POINT('Ctrl Pts',(4.49736521340071,-1.36473368385825,0.676631564755462));
#10461=CARTESIAN_POINT('Ctrl Pts',(8.70006933407556,-1.57940608001781,0.626799670546273));
#10462=CARTESIAN_POINT('Ctrl Pts',(7.3004573192207,-1.49190036240803,0.626879818917698));
#10463=CARTESIAN_POINT('Ctrl Pts',(5.89892183391985,-1.43119871194172,0.62691759730524));
#10464=CARTESIAN_POINT('Ctrl Pts',(4.49670869913724,-1.38441313147668,0.626940642142451));
#10465=CARTESIAN_POINT('Ctrl Pts',(8.7,-1.5805153611151,0.605119933308333));
#10466=CARTESIAN_POINT('Ctrl Pts',(7.30039998287682,-1.49303044794594,0.605214477495697));
#10467=CARTESIAN_POINT('Ctrl Pts',(5.89887670103551,-1.4323384618751,0.605259402637312));
#10468=CARTESIAN_POINT('Ctrl Pts',(4.49667047719213,-1.38555885946567,0.605286598232956));
#10469=CARTESIAN_POINT('Ctrl Pts',(8.70000000036771,-1.48045180452391,0.7));
#10470=CARTESIAN_POINT('Ctrl Pts',(7.30120024114866,-1.39310147361351,0.7));
#10471=CARTESIAN_POINT('Ctrl Pts',(5.90078591724148,-1.332484999384,0.7));
#10472=CARTESIAN_POINT('Ctrl Pts',(4.5,-1.28575421950843,0.7));
#10473=CARTESIAN_POINT('Origin',(6.87409734069396,-2.22251806091942E-16,
0.7));
#10474=CARTESIAN_POINT('Ctrl Pts',(4.5,1.28575421950843,0.7));
#10475=CARTESIAN_POINT('Ctrl Pts',(5.9007859172415,1.332484999384,0.7));
#10476=CARTESIAN_POINT('Ctrl Pts',(7.30120024114871,1.39310147361351,0.7));
#10477=CARTESIAN_POINT('Ctrl Pts',(8.70000000036779,1.48045180452391,0.7));
#10478=CARTESIAN_POINT('Ctrl Pts',(4.5,1.28575421950843,0.7));
#10479=CARTESIAN_POINT('Ctrl Pts',(5.90286553803659,1.3325543763676,0.7));
#10480=CARTESIAN_POINT('Ctrl Pts',(7.30535837857749,1.39328148786737,0.7));
#10481=CARTESIAN_POINT('Ctrl Pts',(8.7062300060629,1.48084102486261,0.7));
#10482=CARTESIAN_POINT('Ctrl Pts',(4.49903600403804,1.314650633636,0.7));
#10483=CARTESIAN_POINT('Ctrl Pts',(5.90170976758769,1.36144968116949,0.700000194339816));
#10484=CARTESIAN_POINT('Ctrl Pts',(7.30392377861185,1.42217417124324,0.699999322371676));
#10485=CARTESIAN_POINT('Ctrl Pts',(8.7044244076592,1.50972892972339,0.7));
#10486=CARTESIAN_POINT('Ctrl Pts',(4.49736521340071,1.36473368385825,0.676631564755462));
#10487=CARTESIAN_POINT('Ctrl Pts',(5.89970879741633,1.41153023905743,0.676622651488038));
#10488=CARTESIAN_POINT('Ctrl Pts',(7.30143307762774,1.47225060169427,0.676608218952397));
#10489=CARTESIAN_POINT('Ctrl Pts',(8.70129509098078,1.55979510296572,0.676577193851887));
#10490=CARTESIAN_POINT('Ctrl Pts',(4.49670869913724,1.38441313147668,0.626940642142451));
#10491=CARTESIAN_POINT('Ctrl Pts',(5.89892183391985,1.43119871194172,0.626917597305239));
#10492=CARTESIAN_POINT('Ctrl Pts',(7.3004573192207,1.49190036240803,0.626879818917698));
#10493=CARTESIAN_POINT('Ctrl Pts',(8.70006933407556,1.57940608001781,0.626799670546273));
#10494=CARTESIAN_POINT('Ctrl Pts',(4.49667047719213,1.38555885946567,0.605286598232956));
#10495=CARTESIAN_POINT('Ctrl Pts',(5.89887670103551,1.4323384618751,0.605259402637312));
#10496=CARTESIAN_POINT('Ctrl Pts',(7.30039998287682,1.49303044794594,0.605214477495697));
#10497=CARTESIAN_POINT('Ctrl Pts',(8.7,1.5805153611151,0.605119933308333));
#10498=CARTESIAN_POINT('Ctrl Pts',(8.7,1.5805153611151,0.605119933308333));
#10499=CARTESIAN_POINT('Ctrl Pts',(7.30150776148394,1.49309969195427,0.605214402664297));
#10500=CARTESIAN_POINT('Ctrl Pts',(5.90109530155974,1.43243455365708,0.605259331490037));
#10501=CARTESIAN_POINT('Ctrl Pts',(4.50000000014037,1.38566996330298,0.605286533623957));
#10502=CARTESIAN_POINT('Ctrl Pts',(4.48978738186405,1.41740792524342,-0.00033019561810394));
#10503=CARTESIAN_POINT('Ctrl Pts',(4.49319153668889,1.40682860198312,0.201542048187577));
#10504=CARTESIAN_POINT('Ctrl Pts',(4.49659574248723,1.39624928130232,0.403414291271564));
#10505=CARTESIAN_POINT('Ctrl Pts',(4.5,1.38566996325095,0.605286533624017));
#10506=CARTESIAN_POINT('Ctrl Pts',(5.89591889571947,1.46411055243784,-0.000276130330627574));
#10507=CARTESIAN_POINT('Ctrl Pts',(5.89707305734581,1.45353136553191,0.201596203762952));
#10508=CARTESIAN_POINT('Ctrl Pts',(5.89822728315404,1.44295217665948,0.403468537584147));
#10509=CARTESIAN_POINT('Ctrl Pts',(5.89938156763751,1.43237299696393,0.605340871133719));
#10510=CARTESIAN_POINT('Ctrl Pts',(7.30266630830786,1.52469223633113,-0.000186944012493549));
#10511=CARTESIAN_POINT('Ctrl Pts',(7.3015714609838,1.51411327886184,0.201685539385503));
#10512=CARTESIAN_POINT('Ctrl Pts',(7.30047669312963,1.50353432123572,0.403558023359145));
#10513=CARTESIAN_POINT('Ctrl Pts',(7.29938199831711,1.49295537435086,0.60543050772214));
#10514=CARTESIAN_POINT('Ctrl Pts',(8.7100201910492,1.61222456240079,1.33887903989646E-6));
#10515=CARTESIAN_POINT('Ctrl Pts',(8.70667727354472,1.60164608969545,0.201874135619353));
#10516=CARTESIAN_POINT('Ctrl Pts',(8.7033344507371,1.59106762573896,0.403746934395602));
#10517=CARTESIAN_POINT('Ctrl Pts',(8.6999917239952,1.58048917070127,0.605619735239495));
#10518=CARTESIAN_POINT('Origin',(4.3,1.48481481481482,0.));
#10519=CARTESIAN_POINT('',(4.3,-1.37908752581626,0.605290299758539));
#10520=CARTESIAN_POINT('Ctrl Pts',(4.3,-1.37908752581626,0.605290299758539));
#10521=CARTESIAN_POINT('Ctrl Pts',(4.3,-1.38444464017247,0.504222347694443));
#10522=CARTESIAN_POINT('Ctrl Pts',(4.3,-1.38980163214303,0.403154389143214));
#10523=CARTESIAN_POINT('Ctrl Pts',(4.3,-1.40049562949383,0.201390955816302));
#10524=CARTESIAN_POINT('Ctrl Pts',(4.3,-1.40583263576898,0.100695481088992));
#10525=CARTESIAN_POINT('Ctrl Pts',(4.3,-1.41116952203211,0.));
#10526=CARTESIAN_POINT('Ctrl Pts',(4.30000000005992,-1.27917501058303,0.7));
#10527=CARTESIAN_POINT('Ctrl Pts',(4.30000000048661,-1.28708628524264,0.699999999884766));
#10528=CARTESIAN_POINT('Ctrl Pts',(4.30000064978116,-1.29493415608545,0.69900616264686));
#10529=CARTESIAN_POINT('Ctrl Pts',(4.30000121018478,-1.30257825621016,0.697119208693397));
#10530=CARTESIAN_POINT('Ctrl Pts',(4.30000152558655,-1.30688044586137,0.696057208766858));
#10531=CARTESIAN_POINT('Ctrl Pts',(4.30000181105247,-1.31111814675806,0.694711271736901));
#10532=CARTESIAN_POINT('Ctrl Pts',(4.30000199036827,-1.31526464671957,0.693092387263961));
#10533=CARTESIAN_POINT('Ctrl Pts',(4.30000231141323,-1.32268849323592,0.690193954859197));
#10534=CARTESIAN_POINT('Ctrl Pts',(4.30000222777046,-1.32973966400828,0.686455190804221));
#10535=CARTESIAN_POINT('Ctrl Pts',(4.30000179417102,-1.33627196700415,0.681957645816867));
#10536=CARTESIAN_POINT('Ctrl Pts',(4.30000155535849,-1.33986974800182,0.679480543652151));
#10537=CARTESIAN_POINT('Ctrl Pts',(4.30000121902461,-1.34330986828215,0.67677238407294));
#10538=CARTESIAN_POINT('Ctrl Pts',(4.30000092191081,-1.34656397897095,0.673841242448196));
#10539=CARTESIAN_POINT('Ctrl Pts',(4.30000063243573,-1.34973442737118,0.670985459666446));
#10540=CARTESIAN_POINT('Ctrl Pts',(4.30000037658882,-1.35270906921767,0.667935271966333));
#10541=CARTESIAN_POINT('Ctrl Pts',(4.30000037869864,-1.35546536049262,0.66470214425512));
#10542=CARTESIAN_POINT('Ctrl Pts',(4.30000038260995,-1.36057515211559,0.658708362304413));
#10543=CARTESIAN_POINT('Ctrl Pts',(4.30000117797282,-1.36493744806469,0.652087250959406));
#10544=CARTESIAN_POINT('Ctrl Pts',(4.30000145944905,-1.36849285270534,0.645004510397983));
#10545=CARTESIAN_POINT('Ctrl Pts',(4.30000148826005,-1.36885677248754,0.644279543857467));
#10546=CARTESIAN_POINT('Ctrl Pts',(4.30000151299237,-1.36921219826683,0.643549721050429));
#10547=CARTESIAN_POINT('Ctrl Pts',(4.30000153317099,-1.36955903781249,0.642815208524159));
#10548=CARTESIAN_POINT('Ctrl Pts',(4.30000173031152,-1.37294758118467,0.635639188419686));
#10549=CARTESIAN_POINT('Ctrl Pts',(4.30000134819424,-1.37548140076902,0.628100134775109));
#10550=CARTESIAN_POINT('Ctrl Pts',(4.30000077902196,-1.37710733725971,0.620366659714886));
#10551=CARTESIAN_POINT('Ctrl Pts',(4.30000041405338,-1.37814993145247,0.615407747584041));
#10552=CARTESIAN_POINT('Ctrl Pts',(4.3,-1.37881837002099,0.610368224776708));
#10553=CARTESIAN_POINT('Ctrl Pts',(4.3,-1.37908752581626,0.605290299758539));
#10554=CARTESIAN_POINT('',(4.3,1.37908752581626,0.605290299758539));
#10555=CARTESIAN_POINT('Ctrl Pts',(4.3,1.37908752581626,0.605290299758539));
#10556=CARTESIAN_POINT('Ctrl Pts',(4.3,1.37866806817032,0.613203837240499));
#10557=CARTESIAN_POINT('Ctrl Pts',(4.30000092021544,1.37728139671899,0.621026590428679));
#10558=CARTESIAN_POINT('Ctrl Pts',(4.30000132151137,1.37501133257008,0.628597948954885));
#10559=CARTESIAN_POINT('Ctrl Pts',(4.30000154544343,1.37374458621782,0.632822935636113));
#10560=CARTESIAN_POINT('Ctrl Pts',(4.30000164013187,1.37220176226583,0.636969676056352));
#10561=CARTESIAN_POINT('Ctrl Pts',(4.30000157305315,1.37039070587839,0.641008268098125));
#10562=CARTESIAN_POINT('Ctrl Pts',(4.30000145288191,1.36714620633991,0.648243387946652));
#10563=CARTESIAN_POINT('Ctrl Pts',(4.30000073948134,1.36307905360626,0.655053358422861));
#10564=CARTESIAN_POINT('Ctrl Pts',(4.3000004635866,1.35825284513469,0.661274801567968));
#10565=CARTESIAN_POINT('Ctrl Pts',(4.30000041199046,1.35735027731582,0.662438297592388));
#10566=CARTESIAN_POINT('Ctrl Pts',(4.30000037986005,1.35642103364291,0.663581140343808));
#10567=CARTESIAN_POINT('Ctrl Pts',(4.30000037943224,1.35546536051643,0.664702144255114));
#10568=CARTESIAN_POINT('Ctrl Pts',(4.300000378582,1.3535659898678,0.666930104702213));
#10569=CARTESIAN_POINT('Ctrl Pts',(4.3000005018795,1.35156225525783,0.669071850305581));
#10570=CARTESIAN_POINT('Ctrl Pts',(4.30000067038034,1.34946148384904,0.671123623013939));
#10571=CARTESIAN_POINT('Ctrl Pts',(4.30000112630012,1.34377733881547,0.676675190215126));
#10572=CARTESIAN_POINT('Ctrl Pts',(4.30000183907902,1.33744971106208,0.68150833207295));
#10573=CARTESIAN_POINT('Ctrl Pts',(4.30000208123143,1.33064243458576,0.685568782013219));
#10574=CARTESIAN_POINT('Ctrl Pts',(4.30000223513396,1.3263159977886,0.688149444058562));
#10575=CARTESIAN_POINT('Ctrl Pts',(4.3000022300233,1.32179485563522,0.690417305529342));
#10576=CARTESIAN_POINT('Ctrl Pts',(4.30000206344016,1.31711540146937,0.692349146556373));
#10577=CARTESIAN_POINT('Ctrl Pts',(4.3000018029167,1.30979708846622,0.695370400063095));
#10578=CARTESIAN_POINT('Ctrl Pts',(4.30000114702936,1.30217656646843,0.69753735975804));
#10579=CARTESIAN_POINT('Ctrl Pts',(4.3000006156201,1.29440092269557,0.69878042986007));
#10580=CARTESIAN_POINT('Ctrl Pts',(4.30000027236218,1.28937833178082,0.699583377215073));
#10581=CARTESIAN_POINT('Ctrl Pts',(4.30000000033581,1.28429042584107,0.69999999992549));
#10582=CARTESIAN_POINT('Ctrl Pts',(4.30000000005992,1.27917501058303,0.7));
#10583=CARTESIAN_POINT('Ctrl Pts',(4.3,1.41116952203211,0.));
#10584=CARTESIAN_POINT('Ctrl Pts',(4.3,1.40583262613343,0.100695662891028));
#10585=CARTESIAN_POINT('Ctrl Pts',(4.3,1.40049561022223,0.201391319421434));
#10586=CARTESIAN_POINT('Ctrl Pts',(4.3,1.38980161287056,0.403154752748307));
#10587=CARTESIAN_POINT('Ctrl Pts',(4.3,1.38444463053604,0.504222529496425));
#10588=CARTESIAN_POINT('Ctrl Pts',(4.3,1.37908752581626,0.605290299758539));
#10589=CARTESIAN_POINT('Ctrl Pts',(4.3,-1.41116952203217,-1.08233907947231E-12));
#10590=CARTESIAN_POINT('Ctrl Pts',(4.30370667985561,-1.40059355144761,0.201807922462111));
#10591=CARTESIAN_POINT('Ctrl Pts',(4.30741340932898,-1.39001758331341,0.403615844144917));
#10592=CARTESIAN_POINT('Ctrl Pts',(4.31112018914117,-1.37944161767694,0.605423765036612));
#10593=CARTESIAN_POINT('Ctrl Pts',(3.22410085073145,-1.37636920007795,-3.90459529712038E-5));
#10594=CARTESIAN_POINT('Ctrl Pts',(3.2295286994181,-1.36579313421488,0.201768811380596));
#10595=CARTESIAN_POINT('Ctrl Pts',(3.23495659078338,-1.35521706809947,0.403576667516588));
#10596=CARTESIAN_POINT('Ctrl Pts',(3.24038452463065,-1.34464100578453,0.605384522622892));
#10597=CARTESIAN_POINT('Ctrl Pts',(2.14856196511704,-1.34935185539723,-5.92140864038068E-5));
#10598=CARTESIAN_POINT('Ctrl Pts',(2.15571155670467,-1.33877574824886,0.201748609775608));
#10599=CARTESIAN_POINT('Ctrl Pts',(2.16286118630165,-1.32819964054015,0.403556432267456));
#10600=CARTESIAN_POINT('Ctrl Pts',(2.17001085376486,-1.31762353633116,0.605364253566666));
#10601=CARTESIAN_POINT('Ctrl Pts',(1.073384157387,-1.32427529283232,-8.86713468529234E-5));
#10602=CARTESIAN_POINT('Ctrl Pts',(1.08225606990756,-1.31369916974321,0.201719104822629));
#10603=CARTESIAN_POINT('Ctrl Pts',(1.09112801825726,-1.30312304798914,0.403526879488275));
#10604=CARTESIAN_POINT('Ctrl Pts',(1.10000000295732,-1.29254692759565,0.605334652628532));
#10605=CARTESIAN_POINT('Ctrl Pts',(1.10000000298281,-1.29254692760111,0.605334652628557));
#10606=CARTESIAN_POINT('Ctrl Pts',(2.16694388170712,-1.31755402957363,0.605319894542965));
#10607=CARTESIAN_POINT('Ctrl Pts',(3.23367147240841,-1.34448060345116,0.605309774863278));
#10608=CARTESIAN_POINT('Ctrl Pts',(4.3,-1.37908752581626,0.605290299758539));
#10609=CARTESIAN_POINT('Ctrl Pts',(4.30323908112369,-1.2792801058419,0.7));
#10610=CARTESIAN_POINT('Ctrl Pts',(3.23565147654712,-1.24463335454069,0.7));
#10611=CARTESIAN_POINT('Ctrl Pts',(2.1678436779024,-1.21768649131741,0.7));
#10612=CARTESIAN_POINT('Ctrl Pts',(1.09999999999999,-1.19266190204553,0.7));
#10613=CARTESIAN_POINT('Ctrl Pts',(4.30230129178181,-1.30817667592415,0.7));
#10614=CARTESIAN_POINT('Ctrl Pts',(3.23485320804887,-1.27353066282864,0.699999860738333));
#10615=CARTESIAN_POINT('Ctrl Pts',(2.16713169816659,-1.24658393122273,0.700000105496227));
#10616=CARTESIAN_POINT('Ctrl Pts',(1.0993228455422,-1.22155728565617,0.7));
#10617=CARTESIAN_POINT('Ctrl Pts',(4.30067574076257,-1.35826558912881,0.676637683834297));
#10618=CARTESIAN_POINT('Ctrl Pts',(3.23346787205668,-1.32362126434549,0.676644071225102));
#10619=CARTESIAN_POINT('Ctrl Pts',(2.16589795861771,-1.29667457247055,0.676647306834711));
#10620=CARTESIAN_POINT('Ctrl Pts',(1.09814906228501,-1.27164470234869,0.676652147774997));
#10621=CARTESIAN_POINT('Ctrl Pts',(4.30003720890047,-1.37794098943329,0.626943772371838));
#10622=CARTESIAN_POINT('Ctrl Pts',(3.23292426239396,-1.34330449078822,0.626960286972675));
#10623=CARTESIAN_POINT('Ctrl Pts',(2.16541285690349,-1.31636171257899,0.6269687859393));
#10624=CARTESIAN_POINT('Ctrl Pts',(1.09768760301306,-1.29133598921902,0.626981304916489));
#10625=CARTESIAN_POINT('Ctrl Pts',(4.3,-1.37908752581626,0.605290299758539));
#10626=CARTESIAN_POINT('Ctrl Pts',(3.23289209128077,-1.34445530919946,0.605309789097661));
#10627=CARTESIAN_POINT('Ctrl Pts',(2.16538453588699,-1.31751467232976,0.605319909330946));
#10628=CARTESIAN_POINT('Ctrl Pts',(1.09766050997011,-1.29249209748956,0.605334684996117));
#10629=CARTESIAN_POINT('Ctrl Pts',(1.09999999999999,1.19266190204553,0.7));
#10630=CARTESIAN_POINT('Ctrl Pts',(2.1678436779024,1.21768649131741,0.7));
#10631=CARTESIAN_POINT('Ctrl Pts',(3.23565147654712,1.24463335454069,0.7));
#10632=CARTESIAN_POINT('Ctrl Pts',(4.30323908112369,1.2792801058419,0.7));
#10633=CARTESIAN_POINT('Ctrl Pts',(1.0993228455422,1.22155728565617,0.7));
#10634=CARTESIAN_POINT('Ctrl Pts',(2.16713169816659,1.24658393122273,0.700000105496227));
#10635=CARTESIAN_POINT('Ctrl Pts',(3.23485320804887,1.27353066282864,0.699999860738333));
#10636=CARTESIAN_POINT('Ctrl Pts',(4.30230129178181,1.30817667592415,0.7));
#10637=CARTESIAN_POINT('Ctrl Pts',(1.09814906228501,1.27164470234869,0.676652147774997));
#10638=CARTESIAN_POINT('Ctrl Pts',(2.16589795861771,1.29667457247055,0.676647306834711));
#10639=CARTESIAN_POINT('Ctrl Pts',(3.23346787205668,1.32362126434549,0.676644071225102));
#10640=CARTESIAN_POINT('Ctrl Pts',(4.30067574076257,1.35826558912881,0.676637683834297));
#10641=CARTESIAN_POINT('Ctrl Pts',(1.09768760301306,1.29133598921902,0.626981304916489));
#10642=CARTESIAN_POINT('Ctrl Pts',(2.16541285690349,1.31636171257899,0.6269687859393));
#10643=CARTESIAN_POINT('Ctrl Pts',(3.23292426239396,1.34330449078822,0.626960286972675));
#10644=CARTESIAN_POINT('Ctrl Pts',(4.30003720890047,1.37794098943329,0.626943772371838));
#10645=CARTESIAN_POINT('Ctrl Pts',(1.09766050997011,1.29249209748956,0.605334684996117));
#10646=CARTESIAN_POINT('Ctrl Pts',(2.16538453588699,1.31751467232976,0.605319909330946));
#10647=CARTESIAN_POINT('Ctrl Pts',(3.23289209128077,1.34445530919946,0.605309789097661));
#10648=CARTESIAN_POINT('Ctrl Pts',(4.3,1.37908752581626,0.605290299758539));
#10649=CARTESIAN_POINT('Ctrl Pts',(4.3,1.37908752581626,0.605290299758539));
#10650=CARTESIAN_POINT('Ctrl Pts',(3.23367147240841,1.34448060345116,0.605309774863278));
#10651=CARTESIAN_POINT('Ctrl Pts',(2.16694388170711,1.31755402957363,0.605319894542965));
#10652=CARTESIAN_POINT('Ctrl Pts',(1.10000000298281,1.29254692760111,0.605334652628557));
#10653=CARTESIAN_POINT('Ctrl Pts',(1.07338415738705,1.32427529283227,-8.86713457716078E-5));
#10654=CARTESIAN_POINT('Ctrl Pts',(1.08225606990759,1.31369916974318,0.201719104823349));
#10655=CARTESIAN_POINT('Ctrl Pts',(1.09112801825728,1.30312304798912,0.403526879488635));
#10656=CARTESIAN_POINT('Ctrl Pts',(1.10000000295732,1.29254692759565,0.605334652628532));
#10657=CARTESIAN_POINT('Ctrl Pts',(2.14856196511707,1.34935185539717,-5.92140853224782E-5));
#10658=CARTESIAN_POINT('Ctrl Pts',(2.15571155670469,1.33877574824882,0.201748609776328));
#10659=CARTESIAN_POINT('Ctrl Pts',(2.16286118630166,1.32819964054013,0.403556432267816));
#10660=CARTESIAN_POINT('Ctrl Pts',(2.17001085376486,1.31762353633116,0.605364253566666));
#10661=CARTESIAN_POINT('Ctrl Pts',(3.22410085073147,1.37636920007789,-3.90459518899617E-5));
#10662=CARTESIAN_POINT('Ctrl Pts',(3.22952869941811,1.36579313421484,0.201768811381317));
#10663=CARTESIAN_POINT('Ctrl Pts',(3.23495659078338,1.35521706809945,0.403576667516948));
#10664=CARTESIAN_POINT('Ctrl Pts',(3.24038452463064,1.34464100578453,0.605384522622892));
#10665=CARTESIAN_POINT('Ctrl Pts',(4.3,1.41116952203211,-1.07899800205757E-15));
#10666=CARTESIAN_POINT('Ctrl Pts',(4.3037066798556,1.40059355144758,0.201807922462832));
#10667=CARTESIAN_POINT('Ctrl Pts',(4.30741340932897,1.39001758331339,0.403615844145277));
#10668=CARTESIAN_POINT('Ctrl Pts',(4.31112018914115,1.37944161767694,0.605423765036611));
#10669=CARTESIAN_POINT('Origin',(0.9,1.39290118819044,0.));
#10670=CARTESIAN_POINT('',(0.900000001878204,-1.28788040994396,0.605337476551879));
#10671=CARTESIAN_POINT('Ctrl Pts',(0.900000001878204,-1.28788040994396,
0.605337476551879));
#10672=CARTESIAN_POINT('Ctrl Pts',(0.900000001878204,-1.29328625806092,
0.504228160928694));
#10673=CARTESIAN_POINT('Ctrl Pts',(0.899999999999999,-1.29869191435855,
0.403118132397745));
#10674=CARTESIAN_POINT('Ctrl Pts',(0.899999999999999,-1.30947917558554,
0.201339438823693));
#10675=CARTESIAN_POINT('Ctrl Pts',(0.9,-1.31486085669789,0.100669384150719));
#10676=CARTESIAN_POINT('Ctrl Pts',(0.9,-1.32024227787037,0.));
#10677=CARTESIAN_POINT('',(0.9,-1.18799600975353,0.7));
#10678=CARTESIAN_POINT('Ctrl Pts',(0.900000000000324,-1.18799600975363,
0.7));
#10679=CARTESIAN_POINT('Ctrl Pts',(0.900000000063601,-1.19590581948314,
0.699999999935493));
#10680=CARTESIAN_POINT('Ctrl Pts',(0.900000451671414,-1.20375274583281,
0.699006541951706));
#10681=CARTESIAN_POINT('Ctrl Pts',(0.900000834722547,-1.21139610511184,
0.697120084132161));
#10682=CARTESIAN_POINT('Ctrl Pts',(0.900001049758257,-1.21568690349652,
0.696061072005504));
#10683=CARTESIAN_POINT('Ctrl Pts',(0.900001241882928,-1.21991360580594,
0.694719604949841));
#10684=CARTESIAN_POINT('Ctrl Pts',(0.900001357948449,-1.22404965357203,
0.693106547509926));
#10685=CARTESIAN_POINT('Ctrl Pts',(0.900001566283472,-1.23147376710855,
0.690211145364658));
#10686=CARTESIAN_POINT('Ctrl Pts',(0.900001483882417,-1.23852542365708,
0.686475281350474));
#10687=CARTESIAN_POINT('Ctrl Pts',(0.90000115772027,-1.24505817055452,0.681980323292531));
#10688=CARTESIAN_POINT('Ctrl Pts',(0.90000097852015,-1.2486473946309,0.67951070187031));
#10689=CARTESIAN_POINT('Ctrl Pts',(0.900000731874511,-1.25207971535834,
0.676811055842604));
#10690=CARTESIAN_POINT('Ctrl Pts',(0.90000051586667,-1.25532695882913,0.673889369778116));
#10691=CARTESIAN_POINT('Ctrl Pts',(0.900000304282776,-1.25850769714062,
0.671027521295527));
#10692=CARTESIAN_POINT('Ctrl Pts',(0.900000119565725,-1.26149151526032,
0.667969976014938));
#10693=CARTESIAN_POINT('Ctrl Pts',(0.900000124706954,-1.26425564062679,
0.664728268702146));
#10694=CARTESIAN_POINT('Ctrl Pts',(0.900000134210909,-1.26936533657602,
0.658735726205464));
#10695=CARTESIAN_POINT('Ctrl Pts',(0.900000724431276,-1.2737272220214,0.652115259198653));
#10696=CARTESIAN_POINT('Ctrl Pts',(0.900000949945503,-1.27728244659665,
0.645033014705304));
#10697=CARTESIAN_POINT('Ctrl Pts',(0.900000972753073,-1.27764200720725,
0.644316745985709));
#10698=CARTESIAN_POINT('Ctrl Pts',(0.900000992743332,-1.27799327761064,
0.64359573459864));
#10699=CARTESIAN_POINT('Ctrl Pts',(0.900001009576454,-1.27833616945273,
0.642870141642621));
#10700=CARTESIAN_POINT('Ctrl Pts',(0.900001176059944,-1.28172744954266,
0.635693858502874));
#10701=CARTESIAN_POINT('Ctrl Pts',(0.900000930108723,-1.28426399347052,
0.628153947608977));
#10702=CARTESIAN_POINT('Ctrl Pts',(0.900000539908504,-1.2858931319598,0.620419547606466));
#10703=CARTESIAN_POINT('Ctrl Pts',(0.900000289636433,-1.28693805157347,
0.615458750034127));
#10704=CARTESIAN_POINT('Ctrl Pts',(0.900000000000001,-1.28760881677759,
0.610417269724172));
#10705=CARTESIAN_POINT('Ctrl Pts',(0.900000000000001,-1.28788040985668,
0.605337476551933));
#10706=CARTESIAN_POINT('',(0.9,1.18799600975353,0.7));
#10707=CARTESIAN_POINT('',(0.9,0.696450594095222,0.7));
#10708=CARTESIAN_POINT('',(0.900000001878204,1.28788040994396,0.605337476551879));
#10709=CARTESIAN_POINT('Ctrl Pts',(0.900000000000001,1.28788040985668,0.605337476551933));
#10710=CARTESIAN_POINT('Ctrl Pts',(0.900000000000001,1.28745726486871,0.613251849878237));
#10711=CARTESIAN_POINT('Ctrl Pts',(0.900000641820462,1.28606767879774,0.621075732439556));
#10712=CARTESIAN_POINT('Ctrl Pts',(0.900000906166769,1.28379497466322,0.628648019961568));
#10713=CARTESIAN_POINT('Ctrl Pts',(0.900001053446495,1.2825287445946,0.632866896498568));
#10714=CARTESIAN_POINT('Ctrl Pts',(0.900001106693909,1.28098738700664,0.637007708770872));
#10715=CARTESIAN_POINT('Ctrl Pts',(0.900001044867119,1.27917862712792,0.641040603354488));
#10716=CARTESIAN_POINT('Ctrl Pts',(0.900000933962191,1.27593407274945,0.64827481168313));
#10717=CARTESIAN_POINT('Ctrl Pts',(0.900000399592996,1.27186725264719,0.655083885116145));
#10718=CARTESIAN_POINT('Ctrl Pts',(0.900000190596867,1.2670411556595,0.661303993035384));
#10719=CARTESIAN_POINT('Ctrl Pts',(0.900000151538061,1.26613921747962,0.662466454716044));
#10720=CARTESIAN_POINT('Ctrl Pts',(0.900000126821978,1.26521063179286,0.663608275427336));
#10721=CARTESIAN_POINT('Ctrl Pts',(0.900000125264574,1.26425564063975,0.664728268702142));
#10722=CARTESIAN_POINT('Ctrl Pts',(0.90000012217056,1.26235840892454,0.66695330163032));
#10723=CARTESIAN_POINT('Ctrl Pts',(0.900000209712012,1.26035699384613,0.66909223571964));
#10724=CARTESIAN_POINT('Ctrl Pts',(0.900000331194293,1.2582587086698,0.671141334714948));
#10725=CARTESIAN_POINT('Ctrl Pts',(0.900000660246931,1.25257519443757,0.676691620936499));
#10726=CARTESIAN_POINT('Ctrl Pts',(0.900001184896248,1.24624785575673,0.681523125886843));
#10727=CARTESIAN_POINT('Ctrl Pts',(0.900001377531805,1.23944073409582,0.685581770965975));
#10728=CARTESIAN_POINT('Ctrl Pts',(0.900001499905572,1.2351164383281,0.68816006802201));
#10729=CARTESIAN_POINT('Ctrl Pts',(0.900001510509735,1.23059756718463,0.690425789971136));
#10730=CARTESIAN_POINT('Ctrl Pts',(0.900001405318139,1.22592052877826,0.692355791713551));
#10731=CARTESIAN_POINT('Ctrl Pts',(0.900001240727996,1.21860250674997,0.695375607682216));
#10732=CARTESIAN_POINT('Ctrl Pts',(0.900000792095824,1.21098234272326,0.697541065921879));
#10733=CARTESIAN_POINT('Ctrl Pts',(0.900000425437202,1.20320741268883,0.698782789564668));
#10734=CARTESIAN_POINT('Ctrl Pts',(0.900000188792485,1.19818940410026,0.699584208982791));
#10735=CARTESIAN_POINT('Ctrl Pts',(0.900000000041206,1.19310633605572,0.699999999958324));
#10736=CARTESIAN_POINT('Ctrl Pts',(0.900000000000325,1.18799600975363,0.7));
#10737=CARTESIAN_POINT('Ctrl Pts',(0.9,1.32024227787037,0.));
#10738=CARTESIAN_POINT('Ctrl Pts',(0.9,1.31486080448354,0.100670360916234));
#10739=CARTESIAN_POINT('Ctrl Pts',(0.9,1.30947907114291,0.201341392534));
#10740=CARTESIAN_POINT('Ctrl Pts',(0.9,1.2986918099064,0.403120086121531));
#10741=CARTESIAN_POINT('Ctrl Pts',(0.900000001878204,1.29328620583358,0.504229137772713));
#10742=CARTESIAN_POINT('Ctrl Pts',(0.900000001878204,1.28788040994396,0.605337476551879));
#10743=CARTESIAN_POINT('Ctrl Pts',(0.899999999999997,-1.32024227787137,
-1.86669707469278E-11));
#10744=CARTESIAN_POINT('Ctrl Pts',(0.909148787559422,-1.30966717532842,
0.201788252636133));
#10745=CARTESIAN_POINT('Ctrl Pts',(0.91829761066914,-1.29909207410335,0.403576503749508));
#10746=CARTESIAN_POINT('Ctrl Pts',(0.92744646984625,-1.28851697422138,0.605364753299354));
#10747=CARTESIAN_POINT('Ctrl Pts',(0.699273108318574,-1.31559634352334,
-5.7001548815619E-6));
#10748=CARTESIAN_POINT('Ctrl Pts',(0.708743431409066,-1.30502123870946,
0.20178254329682));
#10749=CARTESIAN_POINT('Ctrl Pts',(0.718213789763005,-1.2944461351935,0.403570785162392));
#10750=CARTESIAN_POINT('Ctrl Pts',(0.727684183892774,-1.28387103300525,
0.605359025419352));
#10751=CARTESIAN_POINT('Ctrl Pts',(0.498558799217305,-1.31100715552056,
-1.1774619888836E-5));
#10752=CARTESIAN_POINT('Ctrl Pts',(0.508350677965937,-1.30043204942944,
0.201776459055217));
#10753=CARTESIAN_POINT('Ctrl Pts',(0.518142591787393,-1.28985694462582,
0.403564691096996));
#10754=CARTESIAN_POINT('Ctrl Pts',(0.527934541191295,-1.27928184113929,
0.60535292148228));
#10755=CARTESIAN_POINT('Ctrl Pts',(0.29785707328833,-1.3064367443434,-1.84041486642056E-5));
#10756=CARTESIAN_POINT('Ctrl Pts',(0.307970527825607,-1.29586163794,0.20176981888596));
#10757=CARTESIAN_POINT('Ctrl Pts',(0.318084017341356,-1.28528653282298,
0.403558040236175));
#10758=CARTESIAN_POINT('Ctrl Pts',(0.328197542344371,-1.27471142901691,
0.605346259877786));
#10759=CARTESIAN_POINT('',(0.32957180616905,-1.2747428754212,0.605346305703265));
#10760=CARTESIAN_POINT('Ctrl Pts',(0.297857995688647,-1.306435779838,1.57426155444895E-16));
#10761=CARTESIAN_POINT('Ctrl Pts',(0.308429283449307,-1.29587142805659,
0.201782098465301));
#10762=CARTESIAN_POINT('Ctrl Pts',(0.319000553694994,-1.28530712634462,
0.403564200350135));
#10763=CARTESIAN_POINT('Ctrl Pts',(0.329571806169048,-1.2747428754212,0.605346305703266));
#10764=CARTESIAN_POINT('Ctrl Pts',(0.32957180616905,-1.2747428754212,0.605346305703265));
#10765=CARTESIAN_POINT('Ctrl Pts',(0.519721397561595,-1.27909449722757,
0.60534313598158));
#10766=CARTESIAN_POINT('Ctrl Pts',(0.709864288600121,-1.28346276435313,
0.605340219076093));
#10767=CARTESIAN_POINT('Ctrl Pts',(0.900000001879218,-1.28788040990034,
0.605337476551906));
#10768=CARTESIAN_POINT('Ctrl Pts',(0.90231940407953,-1.18804989493878,0.7));
#10769=CARTESIAN_POINT('Ctrl Pts',(0.712166351817731,-1.18363199317816,
0.7));
#10770=CARTESIAN_POINT('Ctrl Pts',(0.522011847238247,-1.17926361631973,
0.7));
#10771=CARTESIAN_POINT('Ctrl Pts',(0.331856371369203,-1.17491202960101,
0.7));
#10772=CARTESIAN_POINT('Ctrl Pts',(0.901648075315333,-1.21694488185794,
0.7));
#10773=CARTESIAN_POINT('Ctrl Pts',(0.711500071980331,-1.21252656425213,
0.69999998041973));
#10774=CARTESIAN_POINT('Ctrl Pts',(0.521348914609444,-1.20815772874132,
0.700000022626678));
#10775=CARTESIAN_POINT('Ctrl Pts',(0.331195161244126,-1.20380556524924,
0.7));
#10776=CARTESIAN_POINT('Ctrl Pts',(0.900484091294294,-1.26704448261357,
0.676664431332699));
#10777=CARTESIAN_POINT('Ctrl Pts',(0.710344780071471,-1.26262550764723,
0.676665329845182));
#10778=CARTESIAN_POINT('Ctrl Pts',(0.520199507967113,-1.25825584722226,
0.676666267597974));
#10779=CARTESIAN_POINT('Ctrl Pts',(0.3300487189482,-1.25390275839508,0.676667306001616));
#10780=CARTESIAN_POINT('Ctrl Pts',(0.90002687589075,-1.28672371253673,0.626983665342106));
#10781=CARTESIAN_POINT('Ctrl Pts',(0.709890987426059,-1.28230548388611,
0.626985988983916));
#10782=CARTESIAN_POINT('Ctrl Pts',(0.519747959090447,-1.27793661492756,
0.626988445273931));
#10783=CARTESIAN_POINT('Ctrl Pts',(0.329598318905021,-1.27358432286302,
0.626991130804315));
#10784=CARTESIAN_POINT('Ctrl Pts',(0.900000001879218,-1.28788040990034,
0.605337476551906));
#10785=CARTESIAN_POINT('Ctrl Pts',(0.709864288600121,-1.28346276435313,
0.605340219076093));
#10786=CARTESIAN_POINT('Ctrl Pts',(0.519721397561595,-1.27909449722757,
0.60534313598158));
#10787=CARTESIAN_POINT('Ctrl Pts',(0.32957180616905,-1.2747428754212,0.605346305703265));
#10788=CARTESIAN_POINT('',(0.331856371369201,-1.17491202962433,0.7));
#10789=CARTESIAN_POINT('Origin',(0.331856371539144,-1.1749120296049,0.6));
#10790=CARTESIAN_POINT('Ctrl Pts',(0.900000000000328,-1.18799600975363,
0.7));
#10791=CARTESIAN_POINT('Ctrl Pts',(0.71062007065371,-1.18359647108512,0.7));
#10792=CARTESIAN_POINT('Ctrl Pts',(0.521238702715143,-1.17924592340069,
0.7));
#10793=CARTESIAN_POINT('Ctrl Pts',(0.331856371369203,-1.17491202960101,
0.7));
#10794=CARTESIAN_POINT('Origin',(6.87409734069396,-2.22251806091942E-16,
0.7));
#10795=CARTESIAN_POINT('',(0.331856371879032,1.17491202961268,0.7));
#10796=CARTESIAN_POINT('',(0.331856371369201,-0.75,0.7));
#10797=CARTESIAN_POINT('Ctrl Pts',(0.331856371879031,1.17491202961268,0.7));
#10798=CARTESIAN_POINT('Ctrl Pts',(0.521238703055026,1.1792459234085,0.7));
#10799=CARTESIAN_POINT('Ctrl Pts',(0.710620070823648,1.18359647108907,0.7));
#10800=CARTESIAN_POINT('Ctrl Pts',(0.900000000000325,1.18799600975363,0.7));
#10801=CARTESIAN_POINT('Ctrl Pts',(0.297857073289265,1.30643674434242,-1.84041299971672E-5));
#10802=CARTESIAN_POINT('Ctrl Pts',(0.30797052782623,1.29586163793935,0.201769818898405));
#10803=CARTESIAN_POINT('Ctrl Pts',(0.318084017341667,1.28528653282265,0.403558040242397));
#10804=CARTESIAN_POINT('Ctrl Pts',(0.328197542344371,1.27471142901691,0.605346259877786));
#10805=CARTESIAN_POINT('Ctrl Pts',(0.49855879921793,1.31100715551957,-1.17746012218085E-5));
#10806=CARTESIAN_POINT('Ctrl Pts',(0.50835067796626,1.30043204942878,0.201776459067662));
#10807=CARTESIAN_POINT('Ctrl Pts',(0.518142591787414,1.28985694462549,0.403564691103219));
#10808=CARTESIAN_POINT('Ctrl Pts',(0.527934541191015,1.27928184113928,0.60535292148228));
#10809=CARTESIAN_POINT('Ctrl Pts',(0.699273108318888,1.31559634352235,-5.70013621459206E-6));
#10810=CARTESIAN_POINT('Ctrl Pts',(0.708743431409089,1.3050212387088,0.201782543309265));
#10811=CARTESIAN_POINT('Ctrl Pts',(0.718213789762737,1.29444613519316,0.403570785168614));
#10812=CARTESIAN_POINT('Ctrl Pts',(0.727684183892215,1.28387103300524,0.605359025419352));
#10813=CARTESIAN_POINT('Ctrl Pts',(0.9,1.32024227787037,-6.93889390390723E-18));
#10814=CARTESIAN_POINT('Ctrl Pts',(0.909148787559144,1.30966717532775,0.201788252648578));
#10815=CARTESIAN_POINT('Ctrl Pts',(0.918297610668582,1.29909207410301,0.403576503755731));
#10816=CARTESIAN_POINT('Ctrl Pts',(0.927446469845411,1.28851697422136,0.605364753299355));
#10817=CARTESIAN_POINT('',(0.329571806169048,1.2747428754212,0.605346305703265));
#10818=CARTESIAN_POINT('Ctrl Pts',(0.900000001879216,1.28788040990034,0.605337476551906));
#10819=CARTESIAN_POINT('Ctrl Pts',(0.709864288600119,1.28346276435313,0.605340219076093));
#10820=CARTESIAN_POINT('Ctrl Pts',(0.519721397561593,1.27909449722757,0.60534313598158));
#10821=CARTESIAN_POINT('Ctrl Pts',(0.329571806169048,1.2747428754212,0.605346305703265));
#10822=CARTESIAN_POINT('Ctrl Pts',(0.329571806169048,1.2747428754212,0.605346305703265));
#10823=CARTESIAN_POINT('Ctrl Pts',(0.319000553694994,1.28530712634462,0.403564200350134));
#10824=CARTESIAN_POINT('Ctrl Pts',(0.308429283449307,1.29587142805659,0.201782098465301));
#10825=CARTESIAN_POINT('Ctrl Pts',(0.297857995688647,1.306435779838,6.03900610074426E-17));
#10826=CARTESIAN_POINT('Ctrl Pts',(0.331856371369201,1.17491202960101,0.7));
#10827=CARTESIAN_POINT('Ctrl Pts',(0.522011847238246,1.17926361631973,0.7));
#10828=CARTESIAN_POINT('Ctrl Pts',(0.712166351817729,1.18363199317816,0.7));
#10829=CARTESIAN_POINT('Ctrl Pts',(0.902319404079528,1.18804989493878,0.7));
#10830=CARTESIAN_POINT('Ctrl Pts',(0.331195161244124,1.20380556524924,0.7));
#10831=CARTESIAN_POINT('Ctrl Pts',(0.521348914609443,1.20815772874132,0.700000022626678));
#10832=CARTESIAN_POINT('Ctrl Pts',(0.711500071980329,1.21252656425213,0.69999998041973));
#10833=CARTESIAN_POINT('Ctrl Pts',(0.901648075315331,1.21694488185794,0.7));
#10834=CARTESIAN_POINT('Ctrl Pts',(0.330048718948197,1.25390275839508,0.676667306001616));
#10835=CARTESIAN_POINT('Ctrl Pts',(0.52019950796711,1.25825584722226,0.676666267597973));
#10836=CARTESIAN_POINT('Ctrl Pts',(0.710344780071469,1.26262550764723,0.676665329845182));
#10837=CARTESIAN_POINT('Ctrl Pts',(0.900484091294292,1.26704448261357,0.676664431332698));
#10838=CARTESIAN_POINT('Ctrl Pts',(0.329598318905018,1.27358432286302,0.626991130804315));
#10839=CARTESIAN_POINT('Ctrl Pts',(0.519747959090446,1.27793661492756,0.62698844527393));
#10840=CARTESIAN_POINT('Ctrl Pts',(0.709890987426057,1.28230548388611,0.626985988983916));
#10841=CARTESIAN_POINT('Ctrl Pts',(0.900026875890748,1.28672371253673,0.626983665342106));
#10842=CARTESIAN_POINT('Ctrl Pts',(0.329571806169048,1.2747428754212,0.605346305703265));
#10843=CARTESIAN_POINT('Ctrl Pts',(0.519721397561593,1.27909449722757,0.60534313598158));
#10844=CARTESIAN_POINT('Ctrl Pts',(0.709864288600119,1.28346276435313,0.605340219076093));
#10845=CARTESIAN_POINT('Ctrl Pts',(0.900000001879216,1.28788040990034,0.605337476551906));
#10846=CARTESIAN_POINT('Origin',(0.331856371369202,1.17491202960101,0.6));
#10847=CARTESIAN_POINT('Origin',(0.331856371369202,1.17491202960101,0.6));
#10848=CARTESIAN_POINT('Origin',(0.331856371369201,1.17491202960879,0.6));
#10849=CARTESIAN_POINT('Origin',(0.331856371369202,1.17491202960101,0.6));
#10850=CARTESIAN_POINT('Origin',(12.8681436286308,1.83274446434879,0.6));
#10851=CARTESIAN_POINT('Origin',(12.8681436286308,1.83274446434879,0.6));
#10852=CARTESIAN_POINT('',(12.9680065821063,1.83274446434879,0.605233595624294));
#10853=CARTESIAN_POINT('Origin',(12.8681436286308,1.83274446434879,0.6));
#10854=CARTESIAN_POINT('Origin',(12.8681436286308,1.83274446434879,0.6));
#10855=CARTESIAN_POINT('Origin',(0.331856371369201,-1.17491202960101,0.6));
#10856=CARTESIAN_POINT('Origin',(0.331856371369201,-1.17491202960101,0.6));
#10857=CARTESIAN_POINT('Origin',(0.331856371369201,-1.17491202960101,0.6));
#10858=CARTESIAN_POINT('Origin',(0.331856371369201,-0.75,0.6));
#10859=CARTESIAN_POINT('Ctrl Pts',(0.297750759617602,-1.30654294555098,
-0.00204689530870639));
#10860=CARTESIAN_POINT('Ctrl Pts',(0.308357792853923,-1.29594287152607,
0.200417501569666));
#10861=CARTESIAN_POINT('Ctrl Pts',(0.318964808457496,-1.28534284790734,
0.40288190189057));
#10862=CARTESIAN_POINT('Ctrl Pts',(0.329571806169048,-1.2747428754212,0.605346305703266));
#10863=CARTESIAN_POINT('Ctrl Pts',(0.268364475985512,-1.30579334864515,
-0.000546070465277405));
#10864=CARTESIAN_POINT('Ctrl Pts',(0.278972236061358,-1.29519218153762,
0.201918231169276));
#10865=CARTESIAN_POINT('Ctrl Pts',(0.289579970322816,-1.28459115545203,
0.404382541571378));
#10866=CARTESIAN_POINT('Ctrl Pts',(0.300187702091134,-1.27399007937578,
0.606846849214128));
#10867=CARTESIAN_POINT('Ctrl Pts',(0.217994620733579,-1.28028753054242,
0.000758348866131992));
#10868=CARTESIAN_POINT('Ctrl Pts',(0.228604439653725,-1.26968580576698,
0.203222517770204));
#10869=CARTESIAN_POINT('Ctrl Pts',(0.239214264875756,-1.259084092946,0.405686686833815));
#10870=CARTESIAN_POINT('Ctrl Pts',(0.24982407554016,-1.24848245399652,0.608150860486448));
#10871=CARTESIAN_POINT('Ctrl Pts',(0.200221638751335,-1.22875730734246,
-0.00100806500432267));
#10872=CARTESIAN_POINT('Ctrl Pts',(0.210832346469089,-1.21815680658782,
0.201456130081263));
#10873=CARTESIAN_POINT('Ctrl Pts',(0.221443027663539,-1.20755634130466,
0.403920328365886));
#10874=CARTESIAN_POINT('Ctrl Pts',(0.232053735729819,-1.1969559383274,0.606384528499152));
#10875=CARTESIAN_POINT('Ctrl Pts',(0.200161316008396,-1.20671181983024,
-0.00215909150772397));
#10876=CARTESIAN_POINT('Ctrl Pts',(0.21077201649647,-1.19611183845239,0.200305134857769));
#10877=CARTESIAN_POINT('Ctrl Pts',(0.221382717124246,-1.18551190812967,
0.402769363888924));
#10878=CARTESIAN_POINT('Ctrl Pts',(0.231993417893744,-1.17491202960101,
0.605233595624295));
#10879=CARTESIAN_POINT('Origin',(12.8681436286308,-1.83274446434879,0.6));
#10880=CARTESIAN_POINT('',(12.9680065821063,-1.83274446434879,0.605233595624295));
#10881=CARTESIAN_POINT('Origin',(12.8681436286308,-1.83274446434879,0.6));
#10882=CARTESIAN_POINT('Origin',(12.8681436286308,-1.83274446434879,0.6));
#10883=CARTESIAN_POINT('Origin',(12.8681436286308,1.1,0.6));
#10884=CARTESIAN_POINT('',(12.9680065821063,1.1,0.605233595624295));
#10885=CARTESIAN_POINT('Ctrl Pts',(12.9998428721614,-1.86475648739599,-0.00223900654757928));
#10886=CARTESIAN_POINT('Ctrl Pts',(12.9892307746816,-1.85408610159386,0.200251876006837));
#10887=CARTESIAN_POINT('Ctrl Pts',(12.9786186779927,-1.84341542867022,0.402742743472647));
#10888=CARTESIAN_POINT('Ctrl Pts',(12.9680065821063,-1.83274446434879,0.605233595624296));
#10889=CARTESIAN_POINT('Ctrl Pts',(12.9997989521977,-1.88070362541494,-0.00140096371806573));
#10890=CARTESIAN_POINT('Ctrl Pts',(12.9891868560404,-1.87003481788623,0.2010900171988));
#10891=CARTESIAN_POINT('Ctrl Pts',(12.9785747412344,-1.85936572080465,0.403580981971657));
#10892=CARTESIAN_POINT('Ctrl Pts',(12.967962646681,-1.84869634914788,0.606071933479074));
#10893=CARTESIAN_POINT('Ctrl Pts',(12.9919061104719,-1.91252097257855,-0.00013797468654593));
#10894=CARTESIAN_POINT('Ctrl Pts',(12.9812924311808,-1.9018552985481,0.202353118580234));
#10895=CARTESIAN_POINT('Ctrl Pts',(12.970678744243,-1.89118929884075,0.404844194499128));
#10896=CARTESIAN_POINT('Ctrl Pts',(12.9600650516023,-1.88052308923615,0.607335259545336));
#10897=CARTESIAN_POINT('Ctrl Pts',(12.9539932318948,-1.95585643963679,0.000158685530800887));
#10898=CARTESIAN_POINT('Ctrl Pts',(12.9433725220626,-1.94519261899951,0.202649549046396));
#10899=CARTESIAN_POINT('Ctrl Pts',(12.9327517623504,-1.93452853669393,0.40514039680648));
#10900=CARTESIAN_POINT('Ctrl Pts',(12.9221309734579,-1.92386419524738,0.607631230057729));
#10901=CARTESIAN_POINT('Ctrl Pts',(12.9129235702791,-1.96658826742031,-0.00142816374191492));
#10902=CARTESIAN_POINT('Ctrl Pts',(12.9022969271978,-1.95592037993921,0.201062184830579));
#10903=CARTESIAN_POINT('Ctrl Pts',(12.891670251582,-1.94525202616943,0.403552507423554));
#10904=CARTESIAN_POINT('Ctrl Pts',(12.8810434760214,-1.93458357684419,0.60604282089977));
#10905=CARTESIAN_POINT('Ctrl Pts',(12.8891437477602,-1.96405813112492,-0.00280773857265357));
#10906=CARTESIAN_POINT('Ctrl Pts',(12.8785151960038,-1.95338599020215,0.199682283294402));
#10907=CARTESIAN_POINT('Ctrl Pts',(12.8678865709412,-1.94271355010484,0.402172286243574));
#10908=CARTESIAN_POINT('Ctrl Pts',(12.8572578715866,-1.93204080633595,0.604662269998931));
#10909=CARTESIAN_POINT('Ctrl Pts',(12.9997255308004,-1.86463850151065,-4.9439619065339E-17));
#10910=CARTESIAN_POINT('Ctrl Pts',(12.9891525471135,-1.85400744222428,0.201744546927532));
#10911=CARTESIAN_POINT('Ctrl Pts',(12.9785795642115,-1.84337609791338,0.403489078876654));
#10912=CARTESIAN_POINT('Ctrl Pts',(12.9680065821063,-1.83274446434879,0.605233595624296));
#10913=CARTESIAN_POINT('Ctrl Pts',(12.8891409639924,1.96405533594058,-0.00275470357795049));
#10914=CARTESIAN_POINT('Ctrl Pts',(12.8785133401458,1.95338412669368,0.199717639954231));
#10915=CARTESIAN_POINT('Ctrl Pts',(12.8678856430057,1.9427126183241,0.402189964571813));
#10916=CARTESIAN_POINT('Ctrl Pts',(12.8572578715866,1.93204080633595,0.604662269998929));
#10917=CARTESIAN_POINT('Ctrl Pts',(12.9049941793403,1.96574209420267,-0.00183498696757459));
#10918=CARTESIAN_POINT('Ctrl Pts',(12.8943678341644,1.95507368670196,0.20063757283533));
#10919=CARTESIAN_POINT('Ctrl Pts',(12.8837414238008,1.94440496992476,0.403110113573296));
#10920=CARTESIAN_POINT('Ctrl Pts',(12.8731149412098,1.93373598667478,0.605582637266155));
#10921=CARTESIAN_POINT('Ctrl Pts',(12.9374710816243,1.9613461313261,-0.000364592700753267));
#10922=CARTESIAN_POINT('Ctrl Pts',(12.9268487371951,1.95068187676899,0.202108391447626));
#10923=CARTESIAN_POINT('Ctrl Pts',(12.9162262930262,1.94001732715406,0.404581355450702));
#10924=CARTESIAN_POINT('Ctrl Pts',(12.9056038462248,1.92935253789361,0.607054307450502));
#10925=CARTESIAN_POINT('Ctrl Pts',(12.9846523118271,1.92834870343354,0.000369250346899581));
#10926=CARTESIAN_POINT('Ctrl Pts',(12.974038022963,1.91768545846127,0.202842678583437));
#10927=CARTESIAN_POINT('Ctrl Pts',(12.9634237233674,1.90702194269714,0.405316092420461));
#10928=CARTESIAN_POINT('Ctrl Pts',(12.9528094065597,1.89635817580376,0.607789492622546));
#10929=CARTESIAN_POINT('Ctrl Pts',(12.9997742127558,1.88867440031858,-0.000928907044737527));
#10930=CARTESIAN_POINT('Ctrl Pts',(12.9891630904765,1.8780073281596,0.201544447891303));
#10931=CARTESIAN_POINT('Ctrl Pts',(12.9785517991681,1.86733992038445,0.404017776344753));
#10932=CARTESIAN_POINT('Ctrl Pts',(12.9679406789684,1.85667229154743,0.606491102406462));
#10933=CARTESIAN_POINT('Ctrl Pts',(12.9998400927033,1.86475369267134,-0.00218597132744988));
#10934=CARTESIAN_POINT('Ctrl Pts',(12.9892289217097,1.85408423839396,0.200287232817622));
#10935=CARTESIAN_POINT('Ctrl Pts',(12.9786177515068,1.84341449704483,0.402760421876702));
#10936=CARTESIAN_POINT('Ctrl Pts',(12.9680065821063,1.83274446434879,0.605233595624294));
#10937=CARTESIAN_POINT('Ctrl Pts',(12.9680065821063,1.83274446434879,0.605233595624294));
#10938=CARTESIAN_POINT('Ctrl Pts',(12.9785795642115,1.84337609791338,0.403489078876654));
#10939=CARTESIAN_POINT('Ctrl Pts',(12.9891525471135,1.85400744222428,0.201744546927532));
#10940=CARTESIAN_POINT('Ctrl Pts',(12.9997255308004,1.86463850151065,1.86916454536501E-16));
#10941=CARTESIAN_POINT('Ctrl Pts',(12.6,1.80383022254432,0.7));
#10942=CARTESIAN_POINT('Ctrl Pts',(12.6893984576578,1.8133105623702,0.7));
#10943=CARTESIAN_POINT('Ctrl Pts',(12.7787800350189,1.82294762441299,0.7));
#10944=CARTESIAN_POINT('Ctrl Pts',(12.8681436286308,1.83274446434879,0.7));
#10945=CARTESIAN_POINT('Ctrl Pts',(12.5969393303222,1.83269196733649,0.7));
#10946=CARTESIAN_POINT('Ctrl Pts',(12.686303642571,1.84217134991284,0.700000098415946));
#10947=CARTESIAN_POINT('Ctrl Pts',(12.7756511334299,1.85180730951691,0.699999896874207));
#10948=CARTESIAN_POINT('Ctrl Pts',(12.8649798835675,1.86160311979107,0.7));
#10949=CARTESIAN_POINT('Ctrl Pts',(12.5916356538948,1.88270499442536,0.67643906321291));
#10950=CARTESIAN_POINT('Ctrl Pts',(12.6809412203008,1.89218243450198,0.676434576658958));
#10951=CARTESIAN_POINT('Ctrl Pts',(12.7702288461642,1.90181652272411,0.676430055978541));
#10952=CARTESIAN_POINT('Ctrl Pts',(12.8594976525144,1.91161025179704,0.676425356750174));
#10953=CARTESIAN_POINT('Ctrl Pts',(12.58957419749,1.90214427893475,0.626447702441804));
#10954=CARTESIAN_POINT('Ctrl Pts',(12.6788572782758,1.91161594713488,0.626436135819418));
#10955=CARTESIAN_POINT('Ctrl Pts',(12.7681225846323,1.92124403769089,0.626424372515079));
#10956=CARTESIAN_POINT('Ctrl Pts',(12.8573684983393,1.93103170500986,0.626412260100396));
#10957=CARTESIAN_POINT('Ctrl Pts',(12.5894662143615,1.90316254677271,0.604704117718382));
#10958=CARTESIAN_POINT('Ctrl Pts',(12.6787484942245,1.91263121188366,0.60469048808123));
#10959=CARTESIAN_POINT('Ctrl Pts',(12.7680127446979,1.92225628370762,0.604676541242762));
#10960=CARTESIAN_POINT('Ctrl Pts',(12.8572578715866,1.93204080633595,0.60466226999893));
#10961=CARTESIAN_POINT('Ctrl Pts',(0.200160815981423,1.20671231935208,-0.00216863259073552));
#10962=CARTESIAN_POINT('Ctrl Pts',(0.21077168314515,1.19611217146534,0.200298774135678));
#10963=CARTESIAN_POINT('Ctrl Pts',(0.221382550448584,1.18551207463533,0.402766183527835));
#10964=CARTESIAN_POINT('Ctrl Pts',(0.231993417893744,1.17491202960101,0.605233595624295));
#10965=CARTESIAN_POINT('Ctrl Pts',(0.200241246305444,1.23610630273461,-0.000633930584249493));
#10966=CARTESIAN_POINT('Ctrl Pts',(0.210852138766318,1.22550544237485,0.201833432539687));
#10967=CARTESIAN_POINT('Ctrl Pts',(0.221462948692539,1.21490467236247,0.404300804744641));
#10968=CARTESIAN_POINT('Ctrl Pts',(0.232073841675177,1.20430390790287,0.60676817279077));
#10969=CARTESIAN_POINT('Ctrl Pts',(0.224595236946023,1.28704077752974,0.000756396927320467));
#10970=CARTESIAN_POINT('Ctrl Pts',(0.235204871724134,1.27643877611169,0.203223757667495));
#10971=CARTESIAN_POINT('Ctrl Pts',(0.245814524913363,1.26583679641595,0.405691118453359));
#10972=CARTESIAN_POINT('Ctrl Pts',(0.256424148042823,1.25523487973404,0.608158484046399));
#10973=CARTESIAN_POINT('Ctrl Pts',(0.275710547013829,1.30598124743532,-0.000930817763883136));
#10974=CARTESIAN_POINT('Ctrl Pts',(0.286318282165364,1.29538020346814,0.201536689442792));
#10975=CARTESIAN_POINT('Ctrl Pts',(0.296926023167072,1.2847792285374,0.404004199876323));
#10976=CARTESIAN_POINT('Ctrl Pts',(0.307533728110612,1.27417827838713,0.606471713336412));
#10977=CARTESIAN_POINT('Ctrl Pts',(0.297750259763447,1.30654344507719,-0.0020564363997533));
#10978=CARTESIAN_POINT('Ctrl Pts',(0.308357459618374,1.29594320454196,0.200411140842193));
#10979=CARTESIAN_POINT('Ctrl Pts',(0.318964641840002,1.28534301441448,0.402878721526778));
#10980=CARTESIAN_POINT('Ctrl Pts',(0.329571806169048,1.2747428754212,0.605346305703265));
#10981=CARTESIAN_POINT('Origin',(13.0002740930491,2.2,-0.0104671912485888));
#10982=CARTESIAN_POINT('Origin',(0.331856371369202,1.17491202960101,0.6));
#10983=CARTESIAN_POINT('',(0.331856371879032,1.17491202961268,0.9));
#10984=CARTESIAN_POINT('',(0.0322675109428289,1.17491202960101,0.615700786872883));
#10985=CARTESIAN_POINT('Origin',(0.331856371369201,1.17491202962433,0.6));
#10986=CARTESIAN_POINT('',(0.325002675768741,1.47440456706157,0.616038917109795));
#10987=CARTESIAN_POINT('Origin',(0.331856371369202,1.17491202960101,0.6));
#10988=CARTESIAN_POINT('Origin',(0.331856371369201,1.17491202960101,0.6));
#10989=CARTESIAN_POINT('Origin',(12.8681436286308,1.83274446434879,0.6));
#10990=CARTESIAN_POINT('',(12.8681436286308,1.83274446434879,0.9));
#10991=CARTESIAN_POINT('',(12.8354863574981,2.13063349031027,0.613986809996789));
#10992=CARTESIAN_POINT('Origin',(12.8681436286308,1.83274446434879,0.6));
#10993=CARTESIAN_POINT('',(13.1677324890572,1.83274446434879,0.615700786872883));
#10994=CARTESIAN_POINT('Origin',(12.8681436286308,1.83274446434879,0.6));
#10995=CARTESIAN_POINT('Origin',(12.8681436286308,1.83274446434879,0.6));
#10996=CARTESIAN_POINT('Origin',(0.331856371369201,-1.17491202960101,0.6));
#10997=CARTESIAN_POINT('',(0.331856371369201,-1.17491202962433,0.9));
#10998=CARTESIAN_POINT('',(0.325002675768743,-1.47440456706157,0.616038917109795));
#10999=CARTESIAN_POINT('Origin',(0.331856371879032,-1.17491202961268,0.6));
#11000=CARTESIAN_POINT('',(0.0322675109428289,-1.17491202960101,0.615700786872884));
#11001=CARTESIAN_POINT('Origin',(0.331856371369201,-1.17491202960101,0.6));
#11002=CARTESIAN_POINT('Origin',(0.331856371369201,-1.17491202960101,0.6));
#11003=CARTESIAN_POINT('Origin',(0.331856371369201,-0.75,0.6));
#11004=CARTESIAN_POINT('',(0.0322675109428289,-0.75,0.615700786872883));
#11005=CARTESIAN_POINT('',(0.331856371369201,-0.75,0.9));
#11006=CARTESIAN_POINT('Ctrl Pts',(0.292429673212981,-1.5069793045954,-0.00614074949474724));
#11007=CARTESIAN_POINT('Ctrl Pts',(0.303287396789886,-1.49612100698918,
0.201252467440773));
#11008=CARTESIAN_POINT('Ctrl Pts',(0.314145064588525,-1.48526276089333,
0.408645689616972));
#11009=CARTESIAN_POINT('Ctrl Pts',(0.325002675768741,-1.47440456706157,
0.616038917109795));
#11010=CARTESIAN_POINT('Ctrl Pts',(0.204270663953122,-1.50473074636003,
-0.00163825452108868));
#11011=CARTESIAN_POINT('Ctrl Pts',(0.215130619942527,-1.49386909866124,
0.205754670272474));
#11012=CARTESIAN_POINT('Ctrl Pts',(0.225990497234893,-1.48300775583971,
0.413147615201549));
#11013=CARTESIAN_POINT('Ctrl Pts',(0.236850363534999,-1.47214617892531,
0.620540547642382));
#11014=CARTESIAN_POINT('Ctrl Pts',(0.0531014592841718,-1.42831231122466,
0.00228331220810075));
#11015=CARTESIAN_POINT('Ctrl Pts',(0.0639677431943945,-1.41744892560022,
0.209675827753147));
#11016=CARTESIAN_POINT('Ctrl Pts',(0.0748340498672138,-1.40658548887187,
0.417068339030394));
#11017=CARTESIAN_POINT('Ctrl Pts',(0.0857003072238147,-1.3957221574093,
0.624460858243749));
#11018=CARTESIAN_POINT('Ctrl Pts',(-0.000158492362241063,-1.27362248439808,
-0.0030242144278773));
#11019=CARTESIAN_POINT('Ctrl Pts',(0.0107105192099893,-1.2627628846508,
0.204368383073371));
#11020=CARTESIAN_POINT('Ctrl Pts',(0.0215794523842628,-1.25190326350425,
0.411760983371354));
#11021=CARTESIAN_POINT('Ctrl Pts',(0.0324484644510542,-1.24104375578019,
0.619153585497454));
#11022=CARTESIAN_POINT('Ctrl Pts',(-0.000339460947516079,-1.20748590713937,
-0.00647730073969574));
#11023=CARTESIAN_POINT('Ctrl Pts',(0.0105295295353408,-1.19662789414299,
0.200915392321314));
#11024=CARTESIAN_POINT('Ctrl Pts',(0.0213985201647323,-1.18576993469886,
0.408308088178364));
#11025=CARTESIAN_POINT('Ctrl Pts',(0.032267510942829,-1.17491202960101,
0.615700786872884));
#11026=CARTESIAN_POINT('Ctrl Pts',(0.292751161823634,-1.50665779898694,
4.33680868994202E-17));
#11027=CARTESIAN_POINT('Ctrl Pts',(0.30350172143464,-1.49590667092872,0.205346300540216));
#11028=CARTESIAN_POINT('Ctrl Pts',(0.314252226354851,-1.48515559337638,
0.410692606218909));
#11029=CARTESIAN_POINT('Ctrl Pts',(0.325002675768741,-1.47440456706157,
0.616038917109795));
#11030=CARTESIAN_POINT('Ctrl Pts',(0.032267510942829,-1.17491202960101,
0.615700786872884));
#11031=CARTESIAN_POINT('Ctrl Pts',(0.021511673816962,-1.18565689645617,
0.410467188483275));
#11032=CARTESIAN_POINT('Ctrl Pts',(0.0107558368367201,-1.19640181653194,
0.205233592872363));
#11033=CARTESIAN_POINT('Ctrl Pts',(-2.19605150036939E-16,-1.20714678905882,
1.11889664200504E-16));
#11034=CARTESIAN_POINT('Origin',(12.8681436286308,-1.83274446434879,0.6));
#11035=CARTESIAN_POINT('',(13.1677324890572,-1.83274446434879,0.615700786872883));
#11036=CARTESIAN_POINT('',(12.8354863574981,-2.13063349031027,0.613986809996789));
#11037=CARTESIAN_POINT('Origin',(12.8681436286308,-1.83274446434879,0.6));
#11038=CARTESIAN_POINT('',(12.8681436286308,-1.83274446434879,0.9));
#11039=CARTESIAN_POINT('Origin',(12.8681436286308,-1.83274446434879,0.6));
#11040=CARTESIAN_POINT('Origin',(12.8681436286308,-1.83274446434879,0.6));
#11041=CARTESIAN_POINT('Origin',(12.8681436286308,1.1,0.6));
#11042=CARTESIAN_POINT('',(13.1677324890572,1.1,0.615700786872883));
#11043=CARTESIAN_POINT('',(12.8681436286308,1.1,0.9));
#11044=CARTESIAN_POINT('Ctrl Pts',(12.8681436286308,-1.83274446434879,0.9));
#11045=CARTESIAN_POINT('Ctrl Pts',(11.0848390724976,-1.63724259846481,0.9));
#11046=CARTESIAN_POINT('Ctrl Pts',(6.90843812479705,-1.33014681916253,0.9));
#11047=CARTESIAN_POINT('Ctrl Pts',(2.72316671642812,-1.22963564084767,0.9));
#11048=CARTESIAN_POINT('Ctrl Pts',(0.331856371369203,-1.17491202960101,
0.9));
#11049=CARTESIAN_POINT('Ctrl Pts',(12.8586523934408,-1.91932043067563,0.9));
#11050=CARTESIAN_POINT('Ctrl Pts',(11.0774332085042,-1.7238803779394,0.89999435405169));
#11051=CARTESIAN_POINT('Ctrl Pts',(6.90489492800773,-1.41683381760594,0.900002805573959));
#11052=CARTESIAN_POINT('Ctrl Pts',(2.72111811994416,-1.31633797570969,0.90000078069347));
#11053=CARTESIAN_POINT('Ctrl Pts',(0.329872740993971,-1.26159263654569,
0.9));
#11054=CARTESIAN_POINT('Ctrl Pts',(12.8422006781022,-2.06938763738452,0.829321796184829));
#11055=CARTESIAN_POINT('Ctrl Pts',(11.0645720435655,-1.87407163985848,0.829602081442736));
#11056=CARTESIAN_POINT('Ctrl Pts',(6.89876476423634,-1.56711486110062,0.829953500700133));
#11057=CARTESIAN_POINT('Ctrl Pts',(2.71756729604702,-1.46664725828863,0.829952661937692));
#11058=CARTESIAN_POINT('Ctrl Pts',(0.326433810179884,-1.41186690836963,
0.829991693349937));
#11059=CARTESIAN_POINT('Ctrl Pts',(12.8358182377562,-2.12760618633201,0.679236780301187));
#11060=CARTESIAN_POINT('Ctrl Pts',(11.0595580661442,-1.93265366192027,0.679962478070753));
#11061=CARTESIAN_POINT('Ctrl Pts',(6.89634818471837,-1.62613750062048,0.680874066334139));
#11062=CARTESIAN_POINT('Ctrl Pts',(2.71617242066404,-1.52567909229178,0.680871998075852));
#11063=CARTESIAN_POINT('Ctrl Pts',(0.325082213976654,-1.47092890938704,
0.680973392412944));
#11064=CARTESIAN_POINT('Ctrl Pts',(12.8354863574981,-2.13063349031027,0.613986809996789));
#11065=CARTESIAN_POINT('Ctrl Pts',(11.0592740266891,-1.93586902238569,0.614841183901826));
#11066=CARTESIAN_POINT('Ctrl Pts',(6.89620783868867,-1.62958780289117,0.615922665333222));
#11067=CARTESIAN_POINT('Ctrl Pts',(2.71609101918193,-1.52912950204849,0.615919334096661));
#11068=CARTESIAN_POINT('Ctrl Pts',(0.325002675768742,-1.47440456706157,
0.616038917109795));
#11069=CARTESIAN_POINT('Ctrl Pts',(0.325002675768742,-1.47440456706157,
0.616038917109795));
#11070=CARTESIAN_POINT('Ctrl Pts',(2.71609101918193,-1.52912950204849,0.615919334096661));
#11071=CARTESIAN_POINT('Ctrl Pts',(6.89620783868867,-1.62958780289117,0.615922665333222));
#11072=CARTESIAN_POINT('Ctrl Pts',(11.0592740266891,-1.93586902238569,0.614841183901826));
#11073=CARTESIAN_POINT('Ctrl Pts',(12.8354863574981,-2.13063349031027,0.613986809996789));
#11074=CARTESIAN_POINT('Ctrl Pts',(12.8681436286308,-1.83274446434879,0.9));
#11075=CARTESIAN_POINT('Ctrl Pts',(11.0848390724976,-1.63724259846481,0.9));
#11076=CARTESIAN_POINT('Ctrl Pts',(6.90843812479705,-1.33014681916253,0.9));
#11077=CARTESIAN_POINT('Ctrl Pts',(2.72316671642812,-1.22963564084767,0.9));
#11078=CARTESIAN_POINT('Ctrl Pts',(0.331856371369203,-1.17491202960101,
0.9));
#11079=CARTESIAN_POINT('Ctrl Pts',(13.2003520234216,-1.86554403325358,-0.00671700702553119));
#11080=CARTESIAN_POINT('Ctrl Pts',(13.1894788444661,-1.85461114646479,0.200755606855839));
#11081=CARTESIAN_POINT('Ctrl Pts',(13.1786056663403,-1.84367795836273,0.40822820490283));
#11082=CARTESIAN_POINT('Ctrl Pts',(13.1677324890572,-1.83274446434879,0.615700786872884));
#11083=CARTESIAN_POINT('Ctrl Pts',(13.200220264666,-1.91338509859121,-0.00420290020003313));
#11084=CARTESIAN_POINT('Ctrl Pts',(13.1893470894366,-1.90245705934317,0.203270015787334));
#11085=CARTESIAN_POINT('Ctrl Pts',(13.1784738563058,-1.89152871992859,0.410742913234898));
#11086=CARTESIAN_POINT('Ctrl Pts',(13.1676006827814,-1.88060011874606,0.61821580043722));
#11087=CARTESIAN_POINT('Ctrl Pts',(13.1765676699515,-2.00888806967359,-0.000409897060868941));
#11088=CARTESIAN_POINT('Ctrl Pts',(13.1656896254949,-1.99796966505382,0.207063364242462));
#11089=CARTESIAN_POINT('Ctrl Pts',(13.1548115799789,-1.98705090404177,0.414536607525659));
#11090=CARTESIAN_POINT('Ctrl Pts',(13.1439334900924,-1.97613202744891,0.622009843787749));
#11091=CARTESIAN_POINT('Ctrl Pts',(13.0627995670833,-2.13884429305335,0.000475886042502645));
#11092=CARTESIAN_POINT('Ctrl Pts',(13.0518999280859,-2.12793157960824,0.207948441605934));
#11093=CARTESIAN_POINT('Ctrl Pts',(13.041000104914,-2.11701865581933,0.415420978499924));
#11094=CARTESIAN_POINT('Ctrl Pts',(13.0301002136907,-2.10610551685206,0.62289350259018));
#11095=CARTESIAN_POINT('Ctrl Pts',(12.9395973356642,-2.17103883395928,-0.00428435975826336));
#11096=CARTESIAN_POINT('Ctrl Pts',(12.9286794517625,-2.16011362679945,0.203186612960554));
#11097=CARTESIAN_POINT('Ctrl Pts',(12.9177614752639,-2.14918756369419,0.410657536673191));
#11098=CARTESIAN_POINT('Ctrl Pts',(12.9068431708026,-2.13826180183499,0.618128462699307));
#11099=CARTESIAN_POINT('Ctrl Pts',(12.8682582931239,-2.16344935299393,-0.00842301254802964));
#11100=CARTESIAN_POINT('Ctrl Pts',(12.857334548107,-2.15251107312608,0.1990469563258));
#11101=CARTESIAN_POINT('Ctrl Pts',(12.8464105706338,-2.1415724540018,0.406516897309109));
#11102=CARTESIAN_POINT('Ctrl Pts',(12.8354863574981,-2.13063349031027,0.61398680999679));
#11103=CARTESIAN_POINT('Ctrl Pts',(13.2,-1.86519007666192,-2.60208521396521E-17));
#11104=CARTESIAN_POINT('Ctrl Pts',(13.1892441622028,-1.85437516893481,0.20523361119958));
#11105=CARTESIAN_POINT('Ctrl Pts',(13.1784883252177,-1.84355996631422,0.410467206902138));
#11106=CARTESIAN_POINT('Ctrl Pts',(13.1677324890572,-1.83274446434879,0.615700786872884));
#11107=CARTESIAN_POINT('Ctrl Pts',(12.8354863574981,-2.13063349031027,0.61398680999679));
#11108=CARTESIAN_POINT('Ctrl Pts',(12.8462627343229,-2.14142441807303,0.409324567403199));
#11109=CARTESIAN_POINT('Ctrl Pts',(12.8570388818204,-2.15221501053143,0.204662297274642));
#11110=CARTESIAN_POINT('Ctrl Pts',(12.8678148030684,-2.16300527278357,2.15973072759112E-16));
#11111=CARTESIAN_POINT('Ctrl Pts',(12.868249917342,2.16344096606744,-0.0082639349430893));
#11112=CARTESIAN_POINT('Ctrl Pts',(12.8573289641336,2.15250548166836,0.19915300804817));
#11113=CARTESIAN_POINT('Ctrl Pts',(12.8464077785869,2.14156965818488,0.406569923163064));
#11114=CARTESIAN_POINT('Ctrl Pts',(12.8354863574981,2.13063349031027,0.613986809996789));
#11115=CARTESIAN_POINT('Ctrl Pts',(12.9158092820513,2.16850062662823,-0.00550483257449158));
#11116=CARTESIAN_POINT('Ctrl Pts',(12.9048922561706,2.15757374897544,0.201912774743134));
#11117=CARTESIAN_POINT('Ctrl Pts',(12.8939750281693,2.14664650750606,0.409330354360154));
#11118=CARTESIAN_POINT('Ctrl Pts',(12.8830575663678,2.13571903132675,0.616747911798467));
#11119=CARTESIAN_POINT('Ctrl Pts',(13.0132876381743,2.15534286385676,-0.00108956416640176));
#11120=CARTESIAN_POINT('Ctrl Pts',(13.002382910411,2.14442874534411,0.206329347217122));
#11121=CARTESIAN_POINT('Ctrl Pts',(12.9914779109393,2.13351435475356,0.413748232116966));
#11122=CARTESIAN_POINT('Ctrl Pts',(12.9805728576194,2.12259976690609,0.621167106093357));
#11123=CARTESIAN_POINT('Ctrl Pts',(13.1547834649542,2.05631410774027,0.001107541479323));
#11124=CARTESIAN_POINT('Ctrl Pts',(13.1439034803964,2.04540309863889,0.208527817346591));
#11125=CARTESIAN_POINT('Ctrl Pts',(13.1330234810862,2.03449182132921,0.415948079627069));
#11126=CARTESIAN_POINT('Ctrl Pts',(13.1221434051731,2.0235803832085,0.623368331037722));
#11127=CARTESIAN_POINT('Ctrl Pts',(13.2001460482598,1.93729725403583,-0.00278676680844524));
#11128=CARTESIAN_POINT('Ctrl Pts',(13.1892758011844,1.92637447722781,0.204633283810596));
#11129=CARTESIAN_POINT('Ctrl Pts',(13.1784050234814,1.91545126126866,0.412053283701094));
#11130=CARTESIAN_POINT('Ctrl Pts',(13.1675347796435,1.9045279459447,0.619473307219386));
#11131=CARTESIAN_POINT('Ctrl Pts',(13.2003436864113,1.86553565046225,-0.00655792739252892));
#11132=CARTESIAN_POINT('Ctrl Pts',(13.1894732864596,1.85460555778322,0.200861659936414));
#11133=CARTESIAN_POINT('Ctrl Pts',(13.1786028873373,1.84367516394377,0.408281231439009));
#11134=CARTESIAN_POINT('Ctrl Pts',(13.1677324890572,1.83274446434879,0.615700786872883));
#11135=CARTESIAN_POINT('Ctrl Pts',(12.8678148030684,2.16300527278357,-3.77302356024956E-17));
#11136=CARTESIAN_POINT('Ctrl Pts',(12.8570388818204,2.15221501053142,0.204662297274639));
#11137=CARTESIAN_POINT('Ctrl Pts',(12.8462627343229,2.14142441807303,0.409324567403198));
#11138=CARTESIAN_POINT('Ctrl Pts',(12.8354863574981,2.13063349031027,0.613986809996789));
#11139=CARTESIAN_POINT('Ctrl Pts',(13.1677324890572,1.83274446434879,0.615700786872883));
#11140=CARTESIAN_POINT('Ctrl Pts',(13.1784883252177,1.84355996631422,0.410467206902138));
#11141=CARTESIAN_POINT('Ctrl Pts',(13.1892441622028,1.85437516893481,0.20523361119958));
#11142=CARTESIAN_POINT('Ctrl Pts',(13.2,1.86519007666192,9.4542429440736E-17));
#11143=CARTESIAN_POINT('Ctrl Pts',(0.3318563713692,1.17491202960101,0.9));
#11144=CARTESIAN_POINT('Ctrl Pts',(2.72316671642811,1.22963564084767,0.9));
#11145=CARTESIAN_POINT('Ctrl Pts',(6.90843812479704,1.33014681916253,0.9));
#11146=CARTESIAN_POINT('Ctrl Pts',(11.0848390724976,1.63724259846481,0.9));
#11147=CARTESIAN_POINT('Ctrl Pts',(12.8681436286308,1.83274446434879,0.9));
#11148=CARTESIAN_POINT('Ctrl Pts',(0.329872740993969,1.26159263654569,0.9));
#11149=CARTESIAN_POINT('Ctrl Pts',(2.72111811994415,1.31633797570969,0.90000078069347));
#11150=CARTESIAN_POINT('Ctrl Pts',(6.90489492800774,1.41683381760594,0.90000280557396));
#11151=CARTESIAN_POINT('Ctrl Pts',(11.0774332085042,1.7238803779394,0.89999435405169));
#11152=CARTESIAN_POINT('Ctrl Pts',(12.8586523934408,1.91932043067563,0.9));
#11153=CARTESIAN_POINT('Ctrl Pts',(0.326433810179882,1.41186690836963,0.829991693349937));
#11154=CARTESIAN_POINT('Ctrl Pts',(2.71756729604703,1.46664725828863,0.829952661937692));
#11155=CARTESIAN_POINT('Ctrl Pts',(6.89876476423633,1.56711486110062,0.829953500700133));
#11156=CARTESIAN_POINT('Ctrl Pts',(11.0645720435655,1.87407163985848,0.829602081442736));
#11157=CARTESIAN_POINT('Ctrl Pts',(12.8422006781022,2.06938763738452,0.829321796184828));
#11158=CARTESIAN_POINT('Ctrl Pts',(0.325082213976652,1.47092890938703,0.680973392412944));
#11159=CARTESIAN_POINT('Ctrl Pts',(2.71617242066403,1.52567909229178,0.680871998075852));
#11160=CARTESIAN_POINT('Ctrl Pts',(6.89634818471838,1.62613750062048,0.680874066334139));
#11161=CARTESIAN_POINT('Ctrl Pts',(11.0595580661442,1.93265366192027,0.679962478070753));
#11162=CARTESIAN_POINT('Ctrl Pts',(12.8358182377562,2.12760618633201,0.679236780301187));
#11163=CARTESIAN_POINT('Ctrl Pts',(0.32500267576874,1.47440456706157,0.616038917109795));
#11164=CARTESIAN_POINT('Ctrl Pts',(2.71609101918192,1.52912950204849,0.615919334096661));
#11165=CARTESIAN_POINT('Ctrl Pts',(6.89620783868868,1.62958780289117,0.615922665333222));
#11166=CARTESIAN_POINT('Ctrl Pts',(11.0592740266891,1.93586902238569,0.614841183901826));
#11167=CARTESIAN_POINT('Ctrl Pts',(12.8354863574981,2.13063349031027,0.613986809996789));
#11168=CARTESIAN_POINT('Ctrl Pts',(12.8354863574981,2.13063349031027,0.613986809996789));
#11169=CARTESIAN_POINT('Ctrl Pts',(11.0592740266891,1.93586902238569,0.614841183901826));
#11170=CARTESIAN_POINT('Ctrl Pts',(6.89620783868868,1.62958780289117,0.615922665333222));
#11171=CARTESIAN_POINT('Ctrl Pts',(2.71609101918192,1.52912950204849,0.615919334096661));
#11172=CARTESIAN_POINT('Ctrl Pts',(0.32500267576874,1.47440456706157,0.616038917109795));
#11173=CARTESIAN_POINT('Ctrl Pts',(0.331856371879031,1.17491202961268,0.900000000000001));
#11174=CARTESIAN_POINT('Ctrl Pts',(2.72316671676804,1.22963564085583,0.9));
#11175=CARTESIAN_POINT('Ctrl Pts',(6.90843812496665,1.330146819175,0.9));
#11176=CARTESIAN_POINT('Ctrl Pts',(11.0848390724976,1.63724259846481,0.9));
#11177=CARTESIAN_POINT('Ctrl Pts',(12.8681436286308,1.83274446434879,0.9));
#11178=CARTESIAN_POINT('Ctrl Pts',(-0.00034095850043725,1.20748740317979,
-0.0065058757516861));
#11179=CARTESIAN_POINT('Ctrl Pts',(0.0105285311667133,1.19662889149835,
0.200896342313063));
#11180=CARTESIAN_POINT('Ctrl Pts',(0.0213980209804115,1.18577043337405,
0.408298563174108));
#11181=CARTESIAN_POINT('Ctrl Pts',(0.0322675109428289,1.17491202960101,
0.615700786872884));
#11182=CARTESIAN_POINT('Ctrl Pts',(-9.96670524854573E-5,1.295669506487,
-0.00190176065173685));
#11183=CARTESIAN_POINT('Ctrl Pts',(0.0107698931059531,1.28480880908357,
0.205500324005663));
#11184=CARTESIAN_POINT('Ctrl Pts',(0.0216392211477595,1.27394827585187,
0.412902429485043));
#11185=CARTESIAN_POINT('Ctrl Pts',(0.0325087822871292,1.26308766450658,
0.62030451837231));
#11186=CARTESIAN_POINT('Ctrl Pts',(0.0728623575603101,1.44853010213391,
0.00227745497540766));
#11187=CARTESIAN_POINT('Ctrl Pts',(0.0837280751164453,1.43766588856392,
0.209679530627308));
#11188=CARTESIAN_POINT('Ctrl Pts',(0.0945938325013454,1.42680163888532,
0.41708160190494));
#11189=CARTESIAN_POINT('Ctrl Pts',(0.105459512942901,1.41593747613444,0.624483681552028));
#11190=CARTESIAN_POINT('Ctrl Pts',(0.226308920038025,1.50529438233544,-0.00279245331904538));
#11191=CARTESIAN_POINT('Ctrl Pts',(0.237168779176494,1.4944331215396,0.204610074087555));
#11192=CARTESIAN_POINT('Ctrl Pts',(0.248028678199983,1.48357195724705,0.412012604182119));
#11193=CARTESIAN_POINT('Ctrl Pts',(0.258888441593434,1.47271077595937,0.619415140009235));
#11194=CARTESIAN_POINT('Ctrl Pts',(0.292428177212438,1.50698080067503,-0.00616932457891824));
#11195=CARTESIAN_POINT('Ctrl Pts',(0.303286399461314,1.49612200437087,0.201233417384176));
#11196=CARTESIAN_POINT('Ctrl Pts',(0.314144565926839,1.48526325958177,0.408636164588429));
#11197=CARTESIAN_POINT('Ctrl Pts',(0.325002675768741,1.47440456706157,0.616038917109795));
#11198=CARTESIAN_POINT('Ctrl Pts',(1.62630325872826E-19,1.20714678905882,
-9.93129189996722E-17));
#11199=CARTESIAN_POINT('Ctrl Pts',(0.0107558368367203,1.19640181653194,
0.205233592872363));
#11200=CARTESIAN_POINT('Ctrl Pts',(0.0215116738169619,1.18565689645617,
0.410467188483274));
#11201=CARTESIAN_POINT('Ctrl Pts',(0.0322675109428289,1.17491202960101,
0.615700786872884));
#11202=CARTESIAN_POINT('Ctrl Pts',(0.325002675768741,1.47440456706157,0.616038917109795));
#11203=CARTESIAN_POINT('Ctrl Pts',(0.314252226354851,1.48515559337638,0.410692606218907));
#11204=CARTESIAN_POINT('Ctrl Pts',(0.30350172143464,1.49590667092872,0.205346300540215));
#11205=CARTESIAN_POINT('Ctrl Pts',(0.292751161823635,1.50665779898694,-1.27502175484295E-16));
#11206=CARTESIAN_POINT('Ctrl Pts',(12.8678148030684,-2.16300527278356,0.));
#11207=CARTESIAN_POINT('Ctrl Pts',(12.8575947095063,-2.15224352891768,0.205346305703265));
#11208=CARTESIAN_POINT('Ctrl Pts',(12.8473746159443,-2.14148178505179,0.41069261140653));
#11209=CARTESIAN_POINT('Ctrl Pts',(12.8371545223823,-2.13072004118591,0.616038917109795));
#11210=CARTESIAN_POINT('Ctrl Pts',(8.67612692265345,-1.70561506876628,0.));
#11211=CARTESIAN_POINT('Ctrl Pts',(8.67274165808153,-1.69485332490039,0.205346305703265));
#11212=CARTESIAN_POINT('Ctrl Pts',(8.66935639350961,-1.68409158103451,0.41069261140653));
#11213=CARTESIAN_POINT('Ctrl Pts',(8.6659711289377,-1.67332983716862,0.616038917109795));
#11214=CARTESIAN_POINT('Ctrl Pts',(4.48443904223854,-1.60211086545473,0.));
#11215=CARTESIAN_POINT('Ctrl Pts',(4.48788860665674,-1.59134912158884,0.205346305703265));
#11216=CARTESIAN_POINT('Ctrl Pts',(4.49133817107494,-1.58058737772296,0.41069261140653));
#11217=CARTESIAN_POINT('Ctrl Pts',(4.49478773549313,-1.56982563385707,0.616038917109795));
#11218=CARTESIAN_POINT('Ctrl Pts',(0.292751161823634,-1.50665779898694,
0.));
#11219=CARTESIAN_POINT('Ctrl Pts',(0.303035555231945,-1.49589605512106,
0.205346305703265));
#11220=CARTESIAN_POINT('Ctrl Pts',(0.313319948640256,-1.48513431125517,
0.41069261140653));
#11221=CARTESIAN_POINT('Ctrl Pts',(0.323604342048567,-1.47437256738929,
0.616038917109795));
#11222=CARTESIAN_POINT('Origin',(0.,-1.5,0.));
#11223=CARTESIAN_POINT('Origin',(6.87409734069396,-2.22044604925031E-16,
0.9));
#11224=CARTESIAN_POINT('Ctrl Pts',(0.292751161823634,1.50665779898694,0.));
#11225=CARTESIAN_POINT('Ctrl Pts',(0.303035555231945,1.49589605512106,0.205346305703265));
#11226=CARTESIAN_POINT('Ctrl Pts',(0.313319948640256,1.48513431125517,0.41069261140653));
#11227=CARTESIAN_POINT('Ctrl Pts',(0.323604342048567,1.47437256738929,0.616038917109795));
#11228=CARTESIAN_POINT('Ctrl Pts',(4.48443904223854,1.60211086545473,0.));
#11229=CARTESIAN_POINT('Ctrl Pts',(4.48788860665674,1.59134912158884,0.205346305703265));
#11230=CARTESIAN_POINT('Ctrl Pts',(4.49133817107493,1.58058737772296,0.41069261140653));
#11231=CARTESIAN_POINT('Ctrl Pts',(4.49478773549313,1.56982563385707,0.616038917109795));
#11232=CARTESIAN_POINT('Ctrl Pts',(8.67612692265345,1.70561506876628,0.));
#11233=CARTESIAN_POINT('Ctrl Pts',(8.67274165808153,1.69485332490039,0.205346305703265));
#11234=CARTESIAN_POINT('Ctrl Pts',(8.66935639350961,1.68409158103451,0.41069261140653));
#11235=CARTESIAN_POINT('Ctrl Pts',(8.66597112893769,1.67332983716862,0.616038917109795));
#11236=CARTESIAN_POINT('Ctrl Pts',(12.8678148030684,2.16300527278356,0.));
#11237=CARTESIAN_POINT('Ctrl Pts',(12.8575947095063,2.15224352891768,0.205346305703265));
#11238=CARTESIAN_POINT('Ctrl Pts',(12.8473746159443,2.14148178505179,0.41069261140653));
#11239=CARTESIAN_POINT('Ctrl Pts',(12.8371545223823,2.13072004118591,0.616038917109795));
#11240=CARTESIAN_POINT('Origin',(13.2,2.2,0.));
#19071=UNCERTAINTY_MEASURE_WITH_UNIT(LENGTH_MEASURE(0.001),#19091,
'DISTANCE_ACCURACY_VALUE',
'Maximum model space distance between geometric entities at asserted c
onnectivities');
#19077=UNCERTAINTY_MEASURE_WITH_UNIT(LENGTH_MEASURE(0.001),#19091,
'DISTANCE_ACCURACY_VALUE',
'Maximum model space distance between geometric entities at asserted c
onnectivities');
#19084=(
GEOMETRIC_REPRESENTATION_CONTEXT(3)
GLOBAL_UNCERTAINTY_ASSIGNED_CONTEXT((#19071))
GLOBAL_UNIT_ASSIGNED_CONTEXT((#19091,#19093,#19094))
REPRESENTATION_CONTEXT('','3D')
);
#19090=(
GEOMETRIC_REPRESENTATION_CONTEXT(3)
GLOBAL_UNCERTAINTY_ASSIGNED_CONTEXT((#19077))
GLOBAL_UNIT_ASSIGNED_CONTEXT((#19091,#19093,#19094))
REPRESENTATION_CONTEXT('','3D')
);
#19091=(
LENGTH_UNIT()
NAMED_UNIT(*)
SI_UNIT(.CENTI.,.METRE.)
);
#19093=(
NAMED_UNIT(*)
PLANE_ANGLE_UNIT()
SI_UNIT($,.RADIAN.)
);
#19094=(
NAMED_UNIT(*)
SI_UNIT($,.STERADIAN.)
SOLID_ANGLE_UNIT()
);
#19101=SHAPE_DEFINITION_REPRESENTATION(#19113,#19141);
#19113=PRODUCT_DEFINITION_SHAPE('',$,#19154);
#19141=SHAPE_REPRESENTATION('',(#7041),#19084);
#19147=PRODUCT_DEFINITION_CONTEXT('part definition',#19185,'design');
#19154=PRODUCT_DEFINITION('2026-11-10-05-09-19-254',
'Upper structural shell',#19166,#19147);
#19166=PRODUCT_DEFINITION_FORMATION('',$,#19193);
#19185=APPLICATION_CONTEXT(
'Core Data for Automotive Mechanical Design Process');
#19186=PRODUCT_CONTEXT('part definition',#19185,'mechanical');
#19193=PRODUCT('2026-11-10-05-09-19-254','Upper structural shell',$,(#19186));
#19203=PRESENTATION_STYLE_ASSIGNMENT((#19211));
#19211=SURFACE_STYLE_USAGE(.BOTH.,#19219);
#19219=SURFACE_SIDE_STYLE('',(#19227));
#19227=SURFACE_STYLE_FILL_AREA(#19235);
#19235=FILL_AREA_STYLE('Structural dark blue',(#19243));
#19243=FILL_AREA_STYLE_COLOUR('Structural dark blue',#19251);
#19251=COLOUR_RGB('Structural dark blue',0.0901960784313725,0.270588235294118,
0.513725490196078);
ENDSEC;
END-ISO-10303-21;
